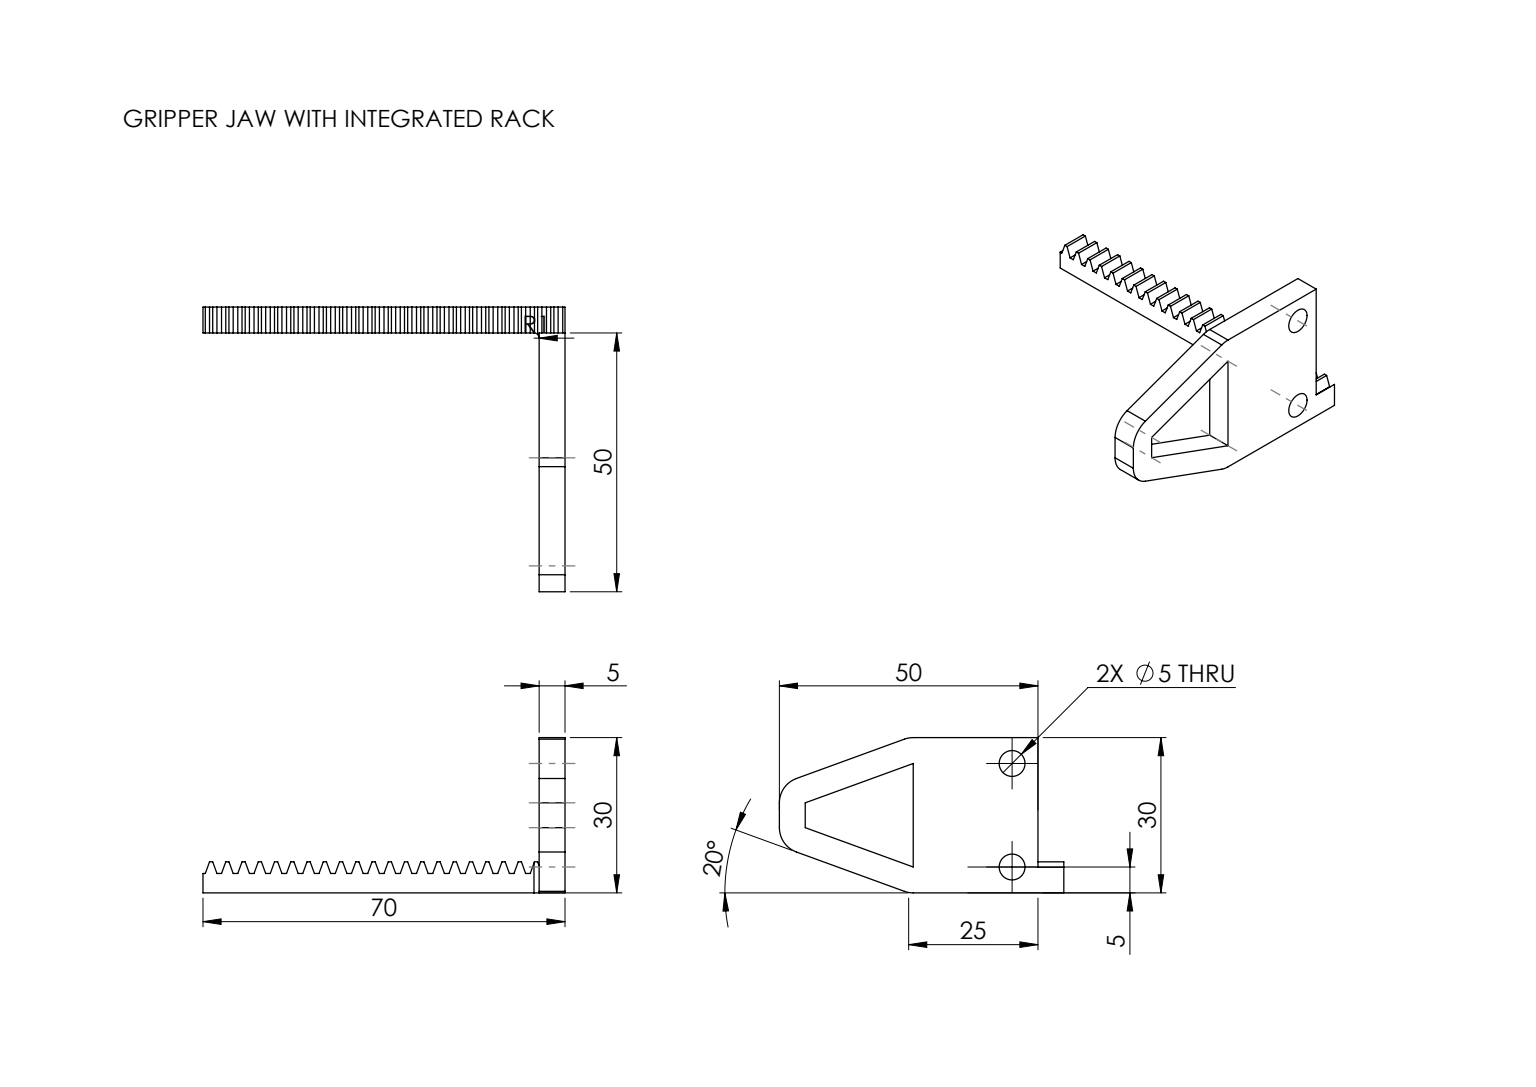
ISO-10303-21;
HEADER;
FILE_DESCRIPTION (('STEP AP214'),
    '1' );
FILE_NAME ('Gripper Jaw with Integrated Rack.step',
    '2026-10-08T13:46:47',
    ( '' ),
    ( '' ),
    'SwSTEP 2.0',
    'SolidWorks 2026',
    '' );
FILE_SCHEMA (( 'AUTOMOTIVE_DESIGN' ));
ENDSEC;

DATA;
#24=FACE_OUTER_BOUND ( 'NONE', #11980, .T. ) ;
#25=VERTEX_POINT ( 'NONE', #5216 ) ;
#26=VECTOR ( 'NONE', #20577, 1000.000000000000114 ) ;
#27=EDGE_CURVE ( 'NONE', #6815, #4177, #10288, .T. ) ;
#28=( GEOMETRIC_REPRESENTATION_CONTEXT ( 3 ) GLOBAL_UNCERTAINTY_ASSIGNED_CONTEXT ( ( #2821 ) ) GLOBAL_UNIT_ASSIGNED_CONTEXT ( ( #14742, #12246, #9459 ) ) REPRESENTATION_CONTEXT ( 'NONE', 'WORKASPACE' ) );
#29=ORIENTED_EDGE ( 'NONE', *, *, #20734, .T. ) ;
#45=ORIENTED_EDGE ( 'NONE', *, *, #7742, .T. ) ;
#53=CARTESIAN_POINT ( 'NONE',  ( 37.82128094071656932, -8.974600000000002353, 5.000000000000079936 ) ) ;
#56=LINE ( 'NONE', #21954, #15596 ) ;
#67=LINE ( 'NONE', #21968, #2877 ) ;
#70=CARTESIAN_POINT ( 'NONE',  ( -15.59503895323380362, -9.000000000000003553, 10.00000000000008882 ) ) ;
#72=ORIENTED_EDGE ( 'NONE', *, *, #3373, .F. ) ;
#76=ORIENTED_EDGE ( 'NONE', *, *, #9529, .F. ) ;
#77=LINE ( 'NONE', #11129, #17930 ) ;
#80=AXIS2_PLACEMENT_3D ( 'NONE', #20688, #15213, #18897 ) ;
#84=CARTESIAN_POINT ( 'NONE',  ( -16.41397198033274307, -11.25000000000000355, 5.000000000000079936 ) ) ;
#86=ORIENTED_EDGE ( 'NONE', *, *, #19557, .T. ) ;
#88=DIRECTION ( 'NONE',  ( 0.3420201433256622181, 0.9396926207859107594, -6.162975822039141593E-32 ) ) ;
#90=PLANE ( 'NONE',  #415 ) ;
#98=LINE ( 'NONE', #14992, #12792 ) ;
#101=DIRECTION ( 'NONE',  ( -0.9396926207859107594, -0.3420201433256623291, 1.540743955509804830E-32 ) ) ;
#102=LINE ( 'NONE', #22483, #7227 ) ;
#104=ORIENTED_EDGE ( 'NONE', *, *, #7323, .T. ) ;
#109=CARTESIAN_POINT ( 'NONE',  ( -1.594879469667249916, -11.25000000000000355, 5.000000000000079936 ) ) ;
#119=EDGE_CURVE ( 'NONE', #21784, #14801, #1618, .T. ) ;
#129=VERTEX_POINT ( 'NONE', #3181 ) ;
#134=DIRECTION ( 'NONE',  ( 0.3420201433256622736, -0.9396926207859106484, -1.232595164407828100E-31 ) ) ;
#138=ORIENTED_EDGE ( 'NONE', *, *, #22563, .F. ) ;
#156=PLANE ( 'NONE',  #640 ) ;
#163=EDGE_LOOP ( 'NONE', ( #11926, #9708, #6526, #4328 ) ) ;
#168=DIRECTION ( 'NONE',  ( 0.3420201433256622181, 0.9396926207859107594, -6.162975822039141593E-32 ) ) ;
#173=AXIS2_PLACEMENT_3D ( 'NONE', #18053, #16495, #3661 ) ;
#174=EDGE_CURVE ( 'NONE', #22879, #11902, #20401, .T. ) ;
#186=DIRECTION ( 'NONE',  ( 1.000000000000000000, 7.703719777548943412E-32, 0.000000000000000000 ) ) ;
#187=DIRECTION ( 'NONE',  ( 0.9396926207859107594, -0.3420201433256623291, 3.697785493223492838E-32 ) ) ;
#195=ORIENTED_EDGE ( 'NONE', *, *, #4034, .T. ) ;
#201=ORIENTED_EDGE ( 'NONE', *, *, #13509, .T. ) ;
#205=CARTESIAN_POINT ( 'NONE',  ( 33.85151041966726382, -11.25000000000000355, 5.000000000000079936 ) ) ;
#214=PRESENTATION_STYLE_ASSIGNMENT (( #11263 ) ) ;
#224=CARTESIAN_POINT ( 'NONE',  ( -19.99999999999999645, -9.000000000000003553, 5.000000000000079936 ) ) ;
#243=ORIENTED_EDGE ( 'NONE', *, *, #7766, .T. ) ;
#248=LINE ( 'NONE', #7582, #20083 ) ;
#270=EDGE_CURVE ( 'NONE', #13563, #6956, #18497, .T. ) ;
#275=ADVANCED_FACE ( 'NONE', ( #14703 ), #22200, .F. ) ;
#279=LINE ( 'NONE', #14812, #13339 ) ;
#280=LINE ( 'NONE', #14938, #18655 ) ;
#284=VECTOR ( 'NONE', #13283, 1000.000000000000000 ) ;
#287=AXIS2_PLACEMENT_3D ( 'NONE', #3170, #5332, #9063 ) ;
#290=FACE_OUTER_BOUND ( 'NONE', #18662, .T. ) ;
#297=VECTOR ( 'NONE', #11394, 1000.000000000000000 ) ;
#306=AXIS2_PLACEMENT_3D ( 'NONE', #17570, #1367, #5089 ) ;
#307=ORIENTED_EDGE ( 'NONE', *, *, #9563, .T. ) ;
#313=VERTEX_POINT ( 'NONE', #3887 ) ;
#327=CARTESIAN_POINT ( 'NONE',  ( 40.13469571966727045, -11.25000000000000355, 10.00000000000008882 ) ) ;
#338=VECTOR ( 'NONE', #6203, 1000.000000000000000 ) ;
#340=CARTESIAN_POINT ( 'NONE',  ( -19.99999999999999645, -9.000000000000003553, 5.000000000000079936 ) ) ;
#345=CARTESIAN_POINT ( 'NONE',  ( -4.471005642132689140, -3.347908285648603766, 10.00000000000008882 ) ) ;
#349=VECTOR ( 'NONE', #3642, 1000.000000000000000 ) ;
#353=PLANE ( 'NONE',  #2572 ) ;
#357=VECTOR ( 'NONE', #88, 1000.000000000000114 ) ;
#369=EDGE_LOOP ( 'NONE', ( #10172, #18701, #9343, #9622 ) ) ;
#371=ORIENTED_EDGE ( 'NONE', *, *, #16704, .T. ) ;
#375=VERTEX_POINT ( 'NONE', #16712 ) ;
#378=VECTOR ( 'NONE', #16810, 1000.000000000000114 ) ;
#379=VECTOR ( 'NONE', #18858, 1000.000000000000000 ) ;
#380=ORIENTED_EDGE ( 'NONE', *, *, #8945, .F. ) ;
#387=ADVANCED_FACE ( 'NONE', ( #290 ), #419, .F. ) ;
#390=CARTESIAN_POINT ( 'NONE',  ( 18.14354716966726144, -11.25000000000000355, 10.00000000000008882 ) ) ;
#394=CARTESIAN_POINT ( 'NONE',  ( 6.625378842019205905, 0.6908453745559488546, 10.00000000000008882 ) ) ;
#397=DIRECTION ( 'NONE',  ( -1.848892746611742040E-32, -0.3420201433256690460, 0.9396926207859083169 ) ) ;
#405=COLOUR_RGB ( '', 0.66274510, 0.83137255, 0.94901961) ;
#415=AXIS2_PLACEMENT_3D ( 'NONE', #22234, #2115, #9450 ) ;
#419=CYLINDRICAL_SURFACE ( 'NONE', #6270, 2.500000000000007550 ) ;
#424=EDGE_CURVE ( 'NONE', #2869, #9385, #10142, .T. ) ;
#432=ORIENTED_EDGE ( 'NONE', *, *, #13078, .F. ) ;
#435=DIRECTION ( 'NONE',  ( -0.9396926207859107594, -0.3420201433256623291, 1.540743955509804830E-32 ) ) ;
#437=DIRECTION ( 'NONE',  ( 1.000000000000000000, 7.703719777548943412E-32, 0.000000000000000000 ) ) ;
#441=EDGE_CURVE ( 'NONE', #4290, #23005, #13728, .T. ) ;
#449=ADVANCED_BREP_SHAPE_REPRESENTATION ( '', ( #22288, #7318 ), #28 ) ;
#452=EDGE_CURVE ( 'NONE', #2752, #12712, #14700, .T. ) ;
#458=EDGE_LOOP ( 'NONE', ( #20331, #17949, #19339, #14429 ) ) ;
#460=DIRECTION ( 'NONE',  ( -7.087422195345011518E-32, -1.000000000000000000, -0.000000000000000000 ) ) ;
#464=DIRECTION ( 'NONE',  ( 0.000000000000000000, 0.000000000000000000, 1.000000000000000000 ) ) ;
#469=ORIENTED_EDGE ( 'NONE', *, *, #19443, .T. ) ;
#470=LINE ( 'NONE', #15224, #23263 ) ;
#472=LINE ( 'NONE', #5983, #26 ) ;
#476=VERTEX_POINT ( 'NONE', #7853 ) ;
#483=CARTESIAN_POINT ( 'NONE',  ( 35.28529930323381336, -9.000000000000001776, 10.00000000000008882 ) ) ;
#487=LINE ( 'NONE', #7810, #20366 ) ;
#496=ORIENTED_EDGE ( 'NONE', *, *, #9040, .T. ) ;
#497=CARTESIAN_POINT ( 'NONE',  ( -19.99999999999999645, -9.000000000000003553, 5.000000000000079936 ) ) ;
#507=CARTESIAN_POINT ( 'NONE',  ( -19.55556463033274284, -11.25000000000000355, 5.000000000000079936 ) ) ;
#513=AXIS2_PLACEMENT_3D ( 'NONE', #21958, #21850, #9422 ) ;
#524=EDGE_CURVE ( 'NONE', #14801, #21630, #9665, .T. ) ;
#525=LINE ( 'NONE', #869, #679 ) ;
#526=PLANE ( 'NONE',  #15257 ) ;
#527=ORIENTED_EDGE ( 'NONE', *, *, #17288, .T. ) ;
#546=EDGE_CURVE ( 'NONE', #10073, #7680, #4255, .T. ) ;
#549=VERTEX_POINT ( 'NONE', #15298 ) ;
#557=ORIENTED_EDGE ( 'NONE', *, *, #22228, .T. ) ;
#561=DIRECTION ( 'NONE',  ( -1.000000000000000000, -7.703719777548943412E-32, 0.000000000000000000 ) ) ;
#563=LINE ( 'NONE', #5844, #11693 ) ;
#564=LINE ( 'NONE', #7663, #15899 ) ;
#575=AXIS2_PLACEMENT_3D ( 'NONE', #18890, #2475, #16877 ) ;
#576=DIRECTION ( 'NONE',  ( 0.3420201433256622181, 0.9396926207859107594, -6.162975822039141593E-32 ) ) ;
#585=EDGE_CURVE ( 'NONE', #18482, #8738, #4962, .T. ) ;
#586=CARTESIAN_POINT ( 'NONE',  ( 118.3095189484530181, -10.00000000000001599, 34.11836509645782201 ) ) ;
#592=VECTOR ( 'NONE', #4754, 1000.000000000000000 ) ;
#595=DIRECTION ( 'NONE',  ( 0.3420201433256622181, 0.9396926207859107594, -6.162975822039141593E-32 ) ) ;
#596=CARTESIAN_POINT ( 'NONE',  ( 32.14370665323380649, -9.000000000000003553, 5.000000000000079936 ) ) ;
#599=CARTESIAN_POINT ( 'NONE',  ( 44.71007725323381976, -9.000000000000003553, 5.000000000000079936 ) ) ;
#601=VECTOR ( 'NONE', #9815, 1000.000000000000000 ) ;
#602=ORIENTED_EDGE ( 'NONE', *, *, #19154, .T. ) ;
#604=EDGE_LOOP ( 'NONE', ( #19723, #19052, #12371, #5086 ) ) ;
#627=ORIENTED_EDGE ( 'NONE', *, *, #11500, .T. ) ;
#633=VERTEX_POINT ( 'NONE', #17729 ) ;
#639=EDGE_CURVE ( 'NONE', #6641, #11647, #14022, .T. ) ;
#640=AXIS2_PLACEMENT_3D ( 'NONE', #3989, #12773, #11329 ) ;
#654=CARTESIAN_POINT ( 'NONE',  ( 7.010965453233809264, -9.000000000000003553, 5.000000000000079936 ) ) ;
#664=CARTESIAN_POINT ( 'NONE',  ( 44.03180068014194148, -9.174246986850796759, 10.00000000000008704 ) ) ;
#672=CARTESIAN_POINT ( 'NONE',  ( 118.3095189484530181, 10.00000000000001599, 12.50000000000002309 ) ) ;
#675=PLANE ( 'NONE',  #14226 ) ;
#679=VECTOR ( 'NONE', #7844, 999.9999999999998863 ) ;
#682=DIRECTION ( 'NONE',  ( 0.3420201433256622181, -0.9396926207859107594, 0.000000000000000000 ) ) ;
#688=ORIENTED_EDGE ( 'NONE', *, *, #7365, .T. ) ;
#689=CARTESIAN_POINT ( 'NONE',  ( 118.3095189484530181, 10.00000000000001599, 34.11836509645782201 ) ) ;
#692=DIRECTION ( 'NONE',  ( 1.000000000000000000, 7.703719777548943412E-32, 0.000000000000000000 ) ) ;
#699=CARTESIAN_POINT ( 'NONE',  ( 40.95362874676621345, -9.000000000000003553, 5.000000000000079936 ) ) ;
#705=ORIENTED_EDGE ( 'NONE', *, *, #16420, .F. ) ;
#714=VECTOR ( 'NONE', #9364, 1000.000000000000000 ) ;
#734=AXIS2_PLACEMENT_3D ( 'NONE', #20200, #14854, #5488 ) ;
#739=AXIS2_PLACEMENT_3D ( 'NONE', #1765, #7059, #9105 ) ;
#746=CARTESIAN_POINT ( 'NONE',  ( -19.99999999999999645, -9.000000000000003553, 5.000000000000079936 ) ) ;
#750=VECTOR ( 'NONE', #3701, 1000.000000000000114 ) ;
#753=EDGE_CURVE ( 'NONE', #22275, #18422, #5493, .T. ) ;
#763=VECTOR ( 'NONE', #682, 1000.000000000000114 ) ;
#785=FACE_OUTER_BOUND ( 'NONE', #1269, .T. ) ;
#788=LINE ( 'NONE', #2452, #19506 ) ;
#796=DIRECTION ( 'NONE',  ( -1.000000000000000000, -7.703719777548943412E-32, 0.000000000000000000 ) ) ;
#813=PLANE ( 'NONE',  #14115 ) ;
#825=DIRECTION ( 'NONE',  ( 1.000000000000000000, 7.703719777548943412E-32, 0.000000000000000000 ) ) ;
#828=LINE ( 'NONE', #8044, #7240 ) ;
#833=ORIENTED_EDGE ( 'NONE', *, *, #15388, .F. ) ;
#842=EDGE_LOOP ( 'NONE', ( #23082, #13876, #7891, #7319, #20724, #21264 ) ) ;
#847=EDGE_LOOP ( 'NONE', ( #5138, #11066, #23192, #10862, #4554, #15889, #19500, #15432, #12929, #23131 ) ) ;
#868=DIRECTION ( 'NONE',  ( 1.000000000000000000, 7.703719777548943412E-32, 0.000000000000000000 ) ) ;
#869=CARTESIAN_POINT ( 'NONE',  ( 50.00000000000000000, -14.69846310392956745, 35.82846581308617573 ) ) ;
#874=ORIENTED_EDGE ( 'NONE', *, *, #14061, .F. ) ;
#877=EDGE_CURVE ( 'NONE', #11647, #2759, #4374, .T. ) ;
#879=ADVANCED_FACE ( 'NONE', ( #785 ), #15426, .F. ) ;
#890=DIRECTION ( 'NONE',  ( 0.000000000000000000, 0.000000000000000000, 1.000000000000000000 ) ) ;
#894=( NAMED_UNIT ( * ) PLANE_ANGLE_UNIT ( ) SI_UNIT ( $, .RADIAN. ) );
#896=ORIENTED_EDGE ( 'NONE', *, *, #11284, .F. ) ;
#902=CARTESIAN_POINT ( 'NONE',  ( 118.3095189484530181, -10.00000000000001954, 12.50000000000002132 ) ) ;
#903=EDGE_CURVE ( 'NONE', #10781, #17912, #2563, .T. ) ;
#915=CARTESIAN_POINT ( 'NONE',  ( 16.42649855928345204, -8.974600000000002353, 5.000000000000079936 ) ) ;
#918=CARTESIAN_POINT ( 'NONE',  ( 50.00000000000000000, 15.00000000000003375, 34.11836509645780069 ) ) ;
#920=EDGE_LOOP ( 'NONE', ( #13456, #4533, #13927, #1880 ) ) ;
#925=CARTESIAN_POINT ( 'NONE',  ( 21.28513981966725765, -11.25000000000000355, 5.000000000000079936 ) ) ;
#926=ORIENTED_EDGE ( 'NONE', *, *, #3827, .F. ) ;
#931=AXIS2_PLACEMENT_3D ( 'NONE', #13447, #6358, #11652 ) ;
#934=CARTESIAN_POINT ( 'NONE',  ( 19.57733605323380743, -9.000000000000001776, 10.00000000000008882 ) ) ;
#938=CARTESIAN_POINT ( 'NONE',  ( -19.55556463033274284, -11.25000000000000355, 10.00000000000008882 ) ) ;
#943=EDGE_CURVE ( 'NONE', #15944, #21012, #11831, .T. ) ;
#944=VECTOR ( 'NONE', #20944, 1000.000000000000114 ) ;
#951=CARTESIAN_POINT ( 'NONE',  ( -19.99999999999999645, -9.000000000000003553, 10.00000000000008882 ) ) ;
#958=EDGE_LOOP ( 'NONE', ( #20659, #18197, #9065, #7020 ) ) ;
#963=VECTOR ( 'NONE', #16673, 1000.000000000000114 ) ;
#964=DIRECTION ( 'NONE',  ( 0.3420201433256622181, 0.9396926207859107594, -6.162975822039141593E-32 ) ) ;
#965=VECTOR ( 'NONE', #15334, 1000.000000000000000 ) ;
#966=LINE ( 'NONE', #19402, #21718 ) ;
#968=CARTESIAN_POINT ( 'NONE',  ( 45.00000000000000000, -10.00000000000001954, 15.00000000000002842 ) ) ;
#974=EDGE_CURVE ( 'NONE', #20062, #17653, #8116, .T. ) ;
#983=VECTOR ( 'NONE', #15941, 1000.000000000000000 ) ;
#1001=EDGE_CURVE ( 'NONE', #4177, #4376, #17325, .T. ) ;
#1014=LINE ( 'NONE', #20885, #4918 ) ;
#1016=VERTEX_POINT ( 'NONE', #2809 ) ;
#1019=LINE ( 'NONE', #13868, #23622 ) ;
#1026=EDGE_LOOP ( 'NONE', ( #16701, #10272, #6399, #3498 ) ) ;
#1035=VERTEX_POINT ( 'NONE', #21709 ) ;
#1041=AXIS2_PLACEMENT_3D ( 'NONE', #5177, #8916, #12519 ) ;
#1045=CARTESIAN_POINT ( 'NONE',  ( -6.170261003233799890, -9.000000000000005329, 10.00000000000008882 ) ) ;
#1051=VECTOR ( 'NONE', #22738, 1000.000000000000000 ) ;
#1052=PLANE ( 'NONE',  #16049 ) ;
#1068=ADVANCED_FACE ( 'NONE', ( #5321 ), #12664, .F. ) ;
#1072=ORIENTED_EDGE ( 'NONE', *, *, #8691, .F. ) ;
#1085=LINE ( 'NONE', #4580, #2998 ) ;
#1106=ORIENTED_EDGE ( 'NONE', *, *, #11011, .F. ) ;
#1110=PLANE ( 'NONE',  #11015 ) ;
#1111=DIRECTION ( 'NONE',  ( -0.9396926207859107594, -0.3420201433256623291, 1.540743955509804830E-32 ) ) ;
#1118=AXIS2_PLACEMENT_3D ( 'NONE', #1736, #20046, #10528 ) ;
#1122=DIRECTION ( 'NONE',  ( 1.000000000000000000, 7.703719777548943412E-32, 0.000000000000000000 ) ) ;
#1124=ORIENTED_EDGE ( 'NONE', *, *, #15503, .T. ) ;
#1126=VERTEX_POINT ( 'NONE', #6891 ) ;
#1129=( GEOMETRIC_REPRESENTATION_CONTEXT ( 3 ) GLOBAL_UNCERTAINTY_ASSIGNED_CONTEXT ( ( #15787 ) ) GLOBAL_UNIT_ASSIGNED_CONTEXT ( ( #16369, #16257, #18157 ) ) REPRESENTATION_CONTEXT ( 'NONE', 'WORKASPACE' ) );
#1131=ORIENTED_EDGE ( 'NONE', *, *, #17544, .F. ) ;
#1134=DIRECTION ( 'NONE',  ( 0.000000000000000000, 0.000000000000000000, 1.000000000000000000 ) ) ;
#1142=VECTOR ( 'NONE', #15800, 1000.000000000000000 ) ;
#1151=CARTESIAN_POINT ( 'NONE',  ( 45.00000000000000000, 10.00000000000001599, 34.11836509645781490 ) ) ;
#1155=DIRECTION ( 'NONE',  ( 0.3420201433256622736, 0.9396926207859106484, 0.000000000000000000 ) ) ;
#1161=MECHANICAL_DESIGN_GEOMETRIC_PRESENTATION_REPRESENTATION('',(#6537),#4181);
#1162=EDGE_CURVE ( 'NONE', #12772, #14872, #1238, .T. ) ;
#1175=VECTOR ( 'NONE', #13412, 1000.000000000000114 ) ;
#1183=PLANE ( 'NONE',  #8483 ) ;
#1186=LINE ( 'NONE', #11771, #12491 ) ;
#1187=DIRECTION ( 'NONE',  ( 0.000000000000000000, 0.000000000000000000, 1.000000000000000000 ) ) ;
#1193=EDGE_LOOP ( 'NONE', ( #2380, #12041, #6105, #18841 ) ) ;
#1194=DIRECTION ( 'NONE',  ( 0.000000000000000000, 0.000000000000000000, -1.000000000000000000 ) ) ;
#1195=ORIENTED_EDGE ( 'NONE', *, *, #7139, .T. ) ;
#1202=EDGE_CURVE ( 'NONE', #10547, #13807, #23402, .T. ) ;
#1204=DIRECTION ( 'NONE',  ( -2.465190328815656418E-32, -0.3420201433256691015, 0.9396926207859083169 ) ) ;
#1211=ORIENTED_EDGE ( 'NONE', *, *, #17544, .T. ) ;
#1216=CARTESIAN_POINT ( 'NONE',  ( 27.56832511966726784, -11.25000000000000355, 5.000000000000079936 ) ) ;
#1218=DIRECTION ( 'NONE',  ( -1.000000000000000000, -7.703719777548943412E-32, 0.000000000000000000 ) ) ;
#1220=AXIS2_PLACEMENT_3D ( 'NONE', #17110, #4292, #7783 ) ;
#1225=LINE ( 'NONE', #8456, #17873 ) ;
#1238=LINE ( 'NONE', #1710, #19369 ) ;
#1240=EDGE_LOOP ( 'NONE', ( #9762, #18516, #602, #12286 ) ) ;
#1249=DIRECTION ( 'NONE',  ( 0.3420201433256622181, 0.9396926207859107594, -6.162975822039141593E-32 ) ) ;
#1251=DIRECTION ( 'NONE',  ( -0.9396926207859107594, -0.3420201433256623291, 1.540743955509804830E-32 ) ) ;
#1254=VECTOR ( 'NONE', #21465, 1000.000000000000000 ) ;
#1269=EDGE_LOOP ( 'NONE', ( #13649, #20440, #1072, #14194, #11128, #20415 ) ) ;
#1290=EDGE_CURVE ( 'NONE', #129, #633, #2063, .T. ) ;
#1298=CARTESIAN_POINT ( 'NONE',  ( -18.73663160323380339, -9.000000000000003553, 5.000000000000079936 ) ) ;
#1300=AXIS2_PLACEMENT_3D ( 'NONE', #4873, #10299, #6568 ) ;
#1302=ADVANCED_FACE ( 'NONE', ( #23641 ), #156, .F. ) ;
#1307=DIRECTION ( 'NONE',  ( -0.3420201433256622181, 0.9396926207859106484, 1.232595164407828100E-31 ) ) ;
#1324=CARTESIAN_POINT ( 'NONE',  ( -10.13078668033273999, -11.25000000000000355, 5.000000000000079936 ) ) ;
#1327=ORIENTED_EDGE ( 'NONE', *, *, #6855, .T. ) ;
#1352=VECTOR ( 'NONE', #12908, 1000.000000000000000 ) ;
#1364=ORIENTED_EDGE ( 'NONE', *, *, #4274, .T. ) ;
#1367=DIRECTION ( 'NONE',  ( -1.000000000000000000, -7.703719777548943412E-32, 0.000000000000000000 ) ) ;
#1370=DIRECTION ( 'NONE',  ( 0.000000000000000000, 0.000000000000000000, -1.000000000000000000 ) ) ;
#1378=LINE ( 'NONE', #19478, #2861 ) ;
#1380=EDGE_LOOP ( 'NONE', ( #22643, #4683, #7458, #15884 ) ) ;
#1383=FACE_OUTER_BOUND ( 'NONE', #10306, .T. ) ;
#1386=CARTESIAN_POINT ( 'NONE',  ( 3.263761790716562139, -8.974600000000002353, 5.000000000000079936 ) ) ;
#1389=DIRECTION ( 'NONE',  ( 1.000000000000000000, 7.703719777548943412E-32, 0.000000000000000000 ) ) ;
#1394=CARTESIAN_POINT ( 'NONE',  ( 28.39650299071657003, -8.974600000000002353, 5.000000000000079936 ) ) ;
#1400=PLANE ( 'NONE',  #4170 ) ;
#1421=ORIENTED_EDGE ( 'NONE', *, *, #7801, .T. ) ;
#1427=EDGE_CURVE ( 'NONE', #12772, #21867, #14168, .T. ) ;
#1433=LINE ( 'NONE', #8656, #7623 ) ;
#1441=FACE_OUTER_BOUND ( 'NONE', #20684, .T. ) ;
#1463=DIRECTION ( 'NONE',  ( -0.3420201433256622181, 0.9396926207859106484, 1.232595164407828100E-31 ) ) ;
#1477=VECTOR ( 'NONE', #3706, 1000.000000000000000 ) ;
#1481=ORIENTED_EDGE ( 'NONE', *, *, #22334, .F. ) ;
#1484=DIRECTION ( 'NONE',  ( 0.3420201433256622736, -0.9396926207859106484, -1.232595164407828100E-31 ) ) ;
#1485=ORIENTED_EDGE ( 'NONE', *, *, #10165, .T. ) ;
#1497=ORIENTED_EDGE ( 'NONE', *, *, #22701, .T. ) ;
#1502=EDGE_CURVE ( 'NONE', #11449, #21785, #7339, .T. ) ;
#1522=ORIENTED_EDGE ( 'NONE', *, *, #14669, .T. ) ;
#1532=CARTESIAN_POINT ( 'NONE',  ( 22.70968385928345157, -8.974600000000002353, 5.000000000000079936 ) ) ;
#1544=EDGE_CURVE ( 'NONE', #8315, #18533, #3361, .T. ) ;
#1547=CARTESIAN_POINT ( 'NONE',  ( 31.53809564071656624, -8.974600000000002353, 10.00000000000008882 ) ) ;
#1550=VERTEX_POINT ( 'NONE', #8895 ) ;
#1558=DIRECTION ( 'NONE',  ( 0.000000000000000000, 0.000000000000000000, 1.000000000000000000 ) ) ;
#1560=LINE ( 'NONE', #9021, #16034 ) ;
#1564=DIRECTION ( 'NONE',  ( 0.3420201433256622181, -0.9396926207859107594, 0.000000000000000000 ) ) ;
#1571=ORIENTED_EDGE ( 'NONE', *, *, #13112, .T. ) ;
#1575=ADVANCED_FACE ( 'NONE', ( #3592 ), #21669, .T. ) ;
#1577=ORIENTED_EDGE ( 'NONE', *, *, #12655, .F. ) ;
#1578=CARTESIAN_POINT ( 'NONE',  ( -18.34148624732256394, -8.396350360904289545, 10.00000000000008882 ) ) ;
#1579=ORIENTED_EDGE ( 'NONE', *, *, #22022, .F. ) ;
#1581=EDGE_LOOP ( 'NONE', ( #527, #11428, #15379, #1485 ) ) ;
#1605=ORIENTED_EDGE ( 'NONE', *, *, #16420, .T. ) ;
#1618=LINE ( 'NONE', #7150, #16240 ) ;
#1629=LINE ( 'NONE', #8603, #18204 ) ;
#1646=FACE_OUTER_BOUND ( 'NONE', #13158, .T. ) ;
#1647=ORIENTED_EDGE ( 'NONE', *, *, #13509, .F. ) ;
#1649=CARTESIAN_POINT ( 'NONE',  ( -19.99999999999999645, -9.000000000000003553, 10.00000000000008882 ) ) ;
#1657=VECTOR ( 'NONE', #15828, 1000.000000000000114 ) ;
#1660=DIRECTION ( 'NONE',  ( 0.000000000000000000, 0.000000000000000000, -1.000000000000000000 ) ) ;
#1667=CARTESIAN_POINT ( 'NONE',  ( 6.396109596766199168, -9.000000000000005329, 10.00000000000008882 ) ) ;
#1669=LINE ( 'NONE', #17740, #23238 ) ;
#1673=LINE ( 'NONE', #21900, #11101 ) ;
#1674=DIRECTION ( 'NONE',  ( 1.000000000000000000, 7.703719777548943412E-32, 0.000000000000000000 ) ) ;
#1679=FACE_OUTER_BOUND ( 'NONE', #7171, .T. ) ;
#1685=ORIENTED_EDGE ( 'NONE', *, *, #1427, .T. ) ;
#1687=EDGE_LOOP ( 'NONE', ( #9119, #10883, #469, #20663 ) ) ;
#1692=EDGE_LOOP ( 'NONE', ( #12643, #19226, #4435, #11190 ) ) ;
#1707=ADVANCED_FACE ( 'NONE', ( #23509 ), #21828, .F. ) ;
#1710=CARTESIAN_POINT ( 'NONE',  ( 43.27628836966725601, -11.25000000000000355, 5.000000000000079936 ) ) ;
#1718=LINE ( 'NONE', #14330, #19683 ) ;
#1721=ORIENTED_EDGE ( 'NONE', *, *, #639, .F. ) ;
#1736=CARTESIAN_POINT ( 'NONE',  ( 46.41788101966725577, -11.25000000000000355, 5.000000000000079936 ) ) ;
#1745=DIRECTION ( 'NONE',  ( -0.9396926207859107594, -0.3420201433256623291, 1.540743955509804830E-32 ) ) ;
#1754=ORIENTED_EDGE ( 'NONE', *, *, #4128, .F. ) ;
#1759=LINE ( 'NONE', #21873, #20990 ) ;
#1763=EDGE_LOOP ( 'NONE', ( #23490, #23359, #7432, #18985 ) ) ;
#1765=CARTESIAN_POINT ( 'NONE',  ( -19.99999999999999645, -9.000000000000003553, 5.000000000000079936 ) ) ;
#1768=DIRECTION ( 'NONE',  ( 7.200064461366508930E-32, 1.000000000000000000, 5.754033390038004481E-16 ) ) ;
#1777=CARTESIAN_POINT ( 'NONE',  ( -19.99999999999999645, -9.000000000000003553, 5.000000000000079936 ) ) ;
#1783=ORIENTED_EDGE ( 'NONE', *, *, #5073, .T. ) ;
#1786=CARTESIAN_POINT ( 'NONE',  ( 45.00000000000000000, -7.098169556225942145, 56.71010071662853136 ) ) ;
#1811=VECTOR ( 'NONE', #23079, 1000.000000000000000 ) ;
#1823=VECTOR ( 'NONE', #6635, 1000.000000000000114 ) ;
#1827=ORIENTED_EDGE ( 'NONE', *, *, #23114, .T. ) ;
#1835=VERTEX_POINT ( 'NONE', #7480 ) ;
#1839=CARTESIAN_POINT ( 'NONE',  ( 27.56832511966726784, -11.25000000000000355, 5.000000000000079936 ) ) ;
#1843=CARTESIAN_POINT ( 'NONE',  ( 45.00000000000000000, -14.69846310392956745, 35.82846581308617573 ) ) ;
#1853=FACE_OUTER_BOUND ( 'NONE', #22121, .T. ) ;
#1856=VERTEX_POINT ( 'NONE', #16932 ) ;
#1859=PLANE ( 'NONE',  #18241 ) ;
#1871=VECTOR ( 'NONE', #9335, 1000.000000000000000 ) ;
#1878=CARTESIAN_POINT ( 'NONE',  ( 118.3095189484530181, 7.098169556225943033, 56.71010071662853136 ) ) ;
#1880=ORIENTED_EDGE ( 'NONE', *, *, #23008, .T. ) ;
#1887=CARTESIAN_POINT ( 'NONE',  ( 32.13446180928345086, -8.974600000000002353, 5.000000000000079936 ) ) ;
#1909=CIRCLE ( 'NONE', #4587, 2.500000000000007550 ) ;
#1935=ADVANCED_FACE ( 'NONE', ( #15270 ), #2532, .F. ) ;
#1942=CARTESIAN_POINT ( 'NONE',  ( 13.29415075323381323, -9.000000000000001776, 5.000000000000079936 ) ) ;
#1948=CARTESIAN_POINT ( 'NONE',  ( 50.00000000000000000, -2.399706452296352932, 60.00000000000021316 ) ) ;
#1956=ORIENTED_EDGE ( 'NONE', *, *, #18593, .T. ) ;
#1959=LINE ( 'NONE', #5447, #11042 ) ;
#1977=LINE ( 'NONE', #5353, #6317 ) ;
#1980=DIRECTION ( 'NONE',  ( 0.000000000000000000, 0.000000000000000000, 1.000000000000000000 ) ) ;
#1981=VERTEX_POINT ( 'NONE', #13582 ) ;
#1989=LINE ( 'NONE', #20550, #20553 ) ;
#1990=EDGE_LOOP ( 'NONE', ( #6524, #5819, #17095, #15250 ) ) ;
#1993=CARTESIAN_POINT ( 'NONE',  ( -3.028668353233801458, -9.000000000000005329, 5.000000000000079936 ) ) ;
#1996=DIRECTION ( 'NONE',  ( 0.000000000000000000, 0.000000000000000000, -1.000000000000000000 ) ) ;
#2004=SURFACE_STYLE_FILL_AREA ( #5852 ) ;
#2021=VECTOR ( 'NONE', #22689, 1000.000000000000000 ) ;
#2037=ADVANCED_FACE ( 'NONE', ( #13351 ), #19066, .T. ) ;
#2040=ORIENTED_EDGE ( 'NONE', *, *, #16782, .T. ) ;
#2043=DIRECTION ( 'NONE',  ( 0.000000000000000000, 0.000000000000000000, 1.000000000000000000 ) ) ;
#2044=VERTEX_POINT ( 'NONE', #6262 ) ;
#2046=CARTESIAN_POINT ( 'NONE',  ( 24.42673246966726452, -11.25000000000000355, 5.000000000000079936 ) ) ;
#2052=PLANE ( 'NONE',  #11510 ) ;
#2060=DIRECTION ( 'NONE',  ( 0.000000000000000000, 0.000000000000000000, 1.000000000000000000 ) ) ;
#2063=LINE ( 'NONE', #14684, #18233 ) ;
#2070=ORIENTED_EDGE ( 'NONE', *, *, #7765, .F. ) ;
#2089=CARTESIAN_POINT ( 'NONE',  ( -9.311853653233802319, -9.000000000000003553, 5.000000000000079936 ) ) ;
#2092=ORIENTED_EDGE ( 'NONE', *, *, #15142, .F. ) ;
#2113=CARTESIAN_POINT ( 'NONE',  ( 0.1129242967662022479, -9.000000000000001776, 10.00000000000008882 ) ) ;
#2115=DIRECTION ( 'NONE',  ( -0.9396926207859107594, -0.3420201433256623291, 1.540743955509804830E-32 ) ) ;
#2116=DIRECTION ( 'NONE',  ( 0.3420201433256622181, -0.9396926207859107594, 0.000000000000000000 ) ) ;
#2128=FACE_OUTER_BOUND ( 'NONE', #8630, .T. ) ;
#2131=VERTEX_POINT ( 'NONE', #3129 ) ;
#2135=CARTESIAN_POINT ( 'NONE',  ( 26.67945438033275707, -11.25000000000000355, 10.00000000000008882 ) ) ;
#2139=LINE ( 'NONE', #4067, #20538 ) ;
#2160=DIRECTION ( 'NONE',  ( 0.000000000000000000, 0.000000000000000000, 1.000000000000000000 ) ) ;
#2196=CARTESIAN_POINT ( 'NONE',  ( 39.24582498033275613, -11.25000000000000355, 10.00000000000008882 ) ) ;
#2197=EDGE_CURVE ( 'NONE', #20481, #6488, #23638, .T. ) ;
#2198=DIRECTION ( 'NONE',  ( -0.3420201433256622181, 0.9396926207859106484, 1.232595164407828100E-31 ) ) ;
#2200=VECTOR ( 'NONE', #14134, 1000.000000000000000 ) ;
#2206=DIRECTION ( 'NONE',  ( 0.000000000000000000, 0.000000000000000000, 1.000000000000000000 ) ) ;
#2207=LINE ( 'NONE', #20162, #379 ) ;
#2229=EDGE_CURVE ( 'NONE', #23499, #10887, #14567, .T. ) ;
#2265=DIRECTION ( 'NONE',  ( 0.3420201433256622181, 0.9396926207859107594, -6.162975822039141593E-32 ) ) ;
#2266=DIRECTION ( 'NONE',  ( 0.3420201433256622736, 0.9396926207859106484, 0.000000000000000000 ) ) ;
#2268=AXIS2_PLACEMENT_3D ( 'NONE', #1394, #16277, #8988 ) ;
#2276=LINE ( 'NONE', #17019, #23504 ) ;
#2284=ORIENTED_EDGE ( 'NONE', *, *, #17458, .F. ) ;
#2286=EDGE_LOOP ( 'NONE', ( #2477, #16579, #11571, #7358 ) ) ;
#2292=ORIENTED_EDGE ( 'NONE', *, *, #13935, .T. ) ;
#2295=ORIENTED_EDGE ( 'NONE', *, *, #5529, .T. ) ;
#2300=VECTOR ( 'NONE', #14417, 1000.000000000000000 ) ;
#2312=DIRECTION ( 'NONE',  ( -7.087422195345011518E-32, -1.000000000000000000, 0.000000000000000000 ) ) ;
#2321=ORIENTED_EDGE ( 'NONE', *, *, #20642, .F. ) ;
#2337=DIRECTION ( 'NONE',  ( 0.000000000000000000, 0.000000000000000000, -1.000000000000000000 ) ) ;
#2345=VERTEX_POINT ( 'NONE', #17498 ) ;
#2354=DIRECTION ( 'NONE',  ( -1.000000000000000000, -7.703719777548943412E-32, 0.000000000000000000 ) ) ;
#2366=VERTEX_POINT ( 'NONE', #13451 ) ;
#2371=EDGE_CURVE ( 'NONE', #14828, #6681, #13805, .T. ) ;
#2374=DIRECTION ( 'NONE',  ( 0.000000000000000000, 0.000000000000000000, -1.000000000000000000 ) ) ;
#2375=DIRECTION ( 'NONE',  ( 1.000000000000000000, 7.703719777548943412E-32, 0.000000000000000000 ) ) ;
#2380=ORIENTED_EDGE ( 'NONE', *, *, #4128, .T. ) ;
#2385=CARTESIAN_POINT ( 'NONE',  ( 40.96287359071656908, -8.974600000000002353, 5.000000000000079936 ) ) ;
#2398=PLANE ( 'NONE',  #23329 ) ;
#2408=VERTEX_POINT ( 'NONE', #13678 ) ;
#2409=ORIENTED_EDGE ( 'NONE', *, *, #10292, .F. ) ;
#2417=DIRECTION ( 'NONE',  ( 0.000000000000000000, 0.000000000000000000, -1.000000000000000000 ) ) ;
#2433=DIRECTION ( 'NONE',  ( 7.087422195345011518E-32, 1.000000000000000000, 0.000000000000000000 ) ) ;
#2444=CARTESIAN_POINT ( 'NONE',  ( 9.537702246766199821, -9.000000000000005329, 5.000000000000079936 ) ) ;
#2448=DIRECTION ( 'NONE',  ( 0.3420201433256622181, -0.9396926207859107594, 0.000000000000000000 ) ) ;
#2452=CARTESIAN_POINT ( 'NONE',  ( 3.869372803233808611, -9.000000000000003553, 5.000000000000079936 ) ) ;
#2457=CARTESIAN_POINT ( 'NONE',  ( 15.00195451966726523, -11.25000000000000355, 5.000000000000079936 ) ) ;
#2461=EDGE_CURVE ( 'NONE', #2366, #11492, #17025, .T. ) ;
#2464=VECTOR ( 'NONE', #9085, 1000.000000000000000 ) ;
#2470=EDGE_CURVE ( 'NONE', #12570, #16559, #7071, .T. ) ;
#2475=DIRECTION ( 'NONE',  ( -0.9396926207859107594, -0.3420201433256623291, 1.540743955509804830E-32 ) ) ;
#2477=ORIENTED_EDGE ( 'NONE', *, *, #19719, .T. ) ;
#2481=DIRECTION ( 'NONE',  ( 1.000000000000000000, 7.703719777548943412E-32, 0.000000000000000000 ) ) ;
#2483=LINE ( 'NONE', #10064, #17040 ) ;
#2486=VECTOR ( 'NONE', #9908, 1000.000000000000000 ) ;
#2523=EDGE_LOOP ( 'NONE', ( #11872, #13867, #11518, #21273 ) ) ;
#2528=EDGE_CURVE ( 'NONE', #4844, #5170, #10805, .T. ) ;
#2532=PLANE ( 'NONE',  #5477 ) ;
#2546=DIRECTION ( 'NONE',  ( -1.000000000000000000, -7.703719777548943412E-32, 0.000000000000000000 ) ) ;
#2547=ORIENTED_EDGE ( 'NONE', *, *, #21664, .F. ) ;
#2556=LINE ( 'NONE', #9904, #5357 ) ;
#2563=LINE ( 'NONE', #9910, #22680 ) ;
#2566=CARTESIAN_POINT ( 'NONE',  ( 118.3095189484530181, 14.69846310392956745, 35.82846581308617573 ) ) ;
#2572=AXIS2_PLACEMENT_3D ( 'NONE', #7687, #15005, #2266 ) ;
#2578=VECTOR ( 'NONE', #1980, 1000.000000000000000 ) ;
#2590=CARTESIAN_POINT ( 'NONE',  ( 50.00000000000000000, -10.00000000000001599, 34.11836509645782201 ) ) ;
#2594=CYLINDRICAL_SURFACE ( 'NONE', #1300, 2.500000000000007550 ) ;
#2598=FACE_OUTER_BOUND ( 'NONE', #23227, .T. ) ;
#2599=LINE ( 'NONE', #19007, #14646 ) ;
#2607=DIRECTION ( 'NONE',  ( 1.000000000000000000, 7.703719777548943412E-32, 0.000000000000000000 ) ) ;
#2611=CARTESIAN_POINT ( 'NONE',  ( 35.27605445928345063, -8.974600000000002353, 5.000000000000079936 ) ) ;
#2618=ORIENTED_EDGE ( 'NONE', *, *, #7801, .F. ) ;
#2620=EDGE_CURVE ( 'NONE', #6127, #11172, #14510, .T. ) ;
#2626=VECTOR ( 'NONE', #4607, 1000.000000000000000 ) ;
#2627=LINE ( 'NONE', #596, #20681 ) ;
#2639=VECTOR ( 'NONE', #1564, 1000.000000000000114 ) ;
#2644=EDGE_CURVE ( 'NONE', #21534, #19492, #98, .T. ) ;
#2658=DIRECTION ( 'NONE',  ( 0.000000000000000000, 0.000000000000000000, 1.000000000000000000 ) ) ;
#2662=VECTOR ( 'NONE', #10669, 1000.000000000000114 ) ;
#2674=VECTOR ( 'NONE', #18506, 1000.000000000000000 ) ;
#2690=VECTOR ( 'NONE', #8286, 1000.000000000000000 ) ;
#2702=VERTEX_POINT ( 'NONE', #12723 ) ;
#2703=DIRECTION ( 'NONE',  ( 0.000000000000000000, 0.000000000000000000, 1.000000000000000000 ) ) ;
#2711=EDGE_LOOP ( 'NONE', ( #2739, #10483, #7158, #19964 ) ) ;
#2714=DIRECTION ( 'NONE',  ( 0.3420201433256622736, -0.9396926207859106484, -1.232595164407828100E-31 ) ) ;
#2724=EDGE_LOOP ( 'NONE', ( #4740, #22610, #2547, #23003 ) ) ;
#2729=VERTEX_POINT ( 'NONE', #5614 ) ;
#2735=DIRECTION ( 'NONE',  ( 7.087422195345011518E-32, 1.000000000000000000, -0.000000000000000000 ) ) ;
#2739=ORIENTED_EDGE ( 'NONE', *, *, #16134, .T. ) ;
#2745=DIRECTION ( 'NONE',  ( 0.000000000000000000, 0.000000000000000000, 1.000000000000000000 ) ) ;
#2752=VERTEX_POINT ( 'NONE', #22117 ) ;
#2756=ORIENTED_EDGE ( 'NONE', *, *, #12561, .F. ) ;
#2759=VERTEX_POINT ( 'NONE', #16522 ) ;
#2763=LINE ( 'NONE', #19179, #20522 ) ;
#2784=VERTEX_POINT ( 'NONE', #9701 ) ;
#2789=DIRECTION ( 'NONE',  ( 0.3420201433256622736, 0.9396926207859106484, 0.000000000000000000 ) ) ;
#2793=ADVANCED_FACE ( 'NONE', ( #13422 ), #15339, .T. ) ;
#2796=EDGE_CURVE ( 'NONE', #10456, #15720, #20343, .T. ) ;
#2809=CARTESIAN_POINT ( 'NONE',  ( 32.96263968033274949, -11.25000000000000355, 5.000000000000079936 ) ) ;
#2814=ORIENTED_EDGE ( 'NONE', *, *, #424, .T. ) ;
#2821=UNCERTAINTY_MEASURE_WITH_UNIT (LENGTH_MEASURE( 1.000000000000000082E-05 ), #14742, 'distance_accuracy_value', 'NONE');
#2824=EDGE_CURVE ( 'NONE', #7050, #8315, #2599, .T. ) ;
#2826=FACE_OUTER_BOUND ( 'NONE', #1763, .T. ) ;
#2834=CARTESIAN_POINT ( 'NONE',  ( -13.27237933033274153, -11.25000000000000355, 5.000000000000079936 ) ) ;
#2837=LINE ( 'NONE', #6576, #23549 ) ;
#2839=DIRECTION ( 'NONE',  ( -0.9396926207859107594, -0.3420201433256623291, 1.540743955509804830E-32 ) ) ;
#2840=ORIENTED_EDGE ( 'NONE', *, *, #174, .T. ) ;
#2856=VECTOR ( 'NONE', #23217, 1000.000000000000000 ) ;
#2857=DIRECTION ( 'NONE',  ( 0.000000000000000000, 0.000000000000000000, 1.000000000000000000 ) ) ;
#2858=ORIENTED_EDGE ( 'NONE', *, *, #16088, .F. ) ;
#2861=VECTOR ( 'NONE', #10419, 1000.000000000000114 ) ;
#2866=DIRECTION ( 'NONE',  ( 0.3420201433256622736, 0.9396926207859106484, 0.000000000000000000 ) ) ;
#2869=VERTEX_POINT ( 'NONE', #16997 ) ;
#2870=LINE ( 'NONE', #20948, #21606 ) ;
#2877=VECTOR ( 'NONE', #4018, 1000.000000000000000 ) ;
#2900=ORIENTED_EDGE ( 'NONE', *, *, #5899, .T. ) ;
#2907=FACE_OUTER_BOUND ( 'NONE', #13297, .T. ) ;
#2914=EDGE_CURVE ( 'NONE', #6569, #13807, #4525, .T. ) ;
#2919=VERTEX_POINT ( 'NONE', #6088 ) ;
#2922=ORIENTED_EDGE ( 'NONE', *, *, #11454, .F. ) ;
#2927=EDGE_LOOP ( 'NONE', ( #23459, #5244, #12916, #5062 ) ) ;
#2933=CARTESIAN_POINT ( 'NONE',  ( -16.41397198033274307, -11.25000000000000355, 5.000000000000079936 ) ) ;
#2934=EDGE_CURVE ( 'NONE', #10781, #21477, #15575, .T. ) ;
#2936=VECTOR ( 'NONE', #23113, 1000.000000000000000 ) ;
#2947=CARTESIAN_POINT ( 'NONE',  ( -8.696997796766190447, -9.000000000000005329, 10.00000000000008882 ) ) ;
#2955=ADVANCED_FACE ( 'NONE', ( #21031 ), #19245, .F. ) ;
#2959=EDGE_LOOP ( 'NONE', ( #76, #17152, #20067, #4280 ) ) ;
#2963=VECTOR ( 'NONE', #21400, 1000.000000000000000 ) ;
#2964=CARTESIAN_POINT ( 'NONE',  ( 50.00000000000000000, 10.00000000000001599, 34.11836509645782201 ) ) ;
#2996=PRODUCT_DEFINITION ( 'UNKNOWN', '', #17578, #4530 ) ;
#2998=VECTOR ( 'NONE', #12138, 1000.000000000000000 ) ;
#3018=ORIENTED_EDGE ( 'NONE', *, *, #14669, .F. ) ;
#3047=CARTESIAN_POINT ( 'NONE',  ( 0.1221691407165617638, -8.974600000000002353, 5.000000000000079936 ) ) ;
#3051=( NAMED_UNIT ( * ) SI_UNIT ( $, .STERADIAN. ) SOLID_ANGLE_UNIT ( ) );
#3052=VECTOR ( 'NONE', #20998, 1000.000000000000000 ) ;
#3054=ORIENTED_EDGE ( 'NONE', *, *, #6171, .F. ) ;
#3067=VECTOR ( 'NONE', #19537, 1000.000000000000000 ) ;
#3081=CARTESIAN_POINT ( 'NONE',  ( 40.13469571966727045, -11.25000000000000355, 5.000000000000079936 ) ) ;
#3083=VECTOR ( 'NONE', #13544, 1000.000000000000000 ) ;
#3090=ORIENTED_EDGE ( 'NONE', *, *, #3478, .T. ) ;
#3111=CARTESIAN_POINT ( 'NONE',  ( 0.000000000000000000, 0.000000000000000000, 0.000000000000000000 ) ) ;
#3118=ORIENTED_EDGE ( 'NONE', *, *, #10409, .F. ) ;
#3120=EDGE_LOOP ( 'NONE', ( #8165, #22127, #18181, #17207 ) ) ;
#3122=CARTESIAN_POINT ( 'NONE',  ( 0.1221691407165617638, -8.974600000000002353, 10.00000000000008882 ) ) ;
#3128=ADVANCED_FACE ( 'NONE', ( #1383 ), #16030, .F. ) ;
#3129=CARTESIAN_POINT ( 'NONE',  ( 28.38725814676620018, -9.000000000000007105, 10.00000000000008882 ) ) ;
#3132=CARTESIAN_POINT ( 'NONE',  ( 45.00000000000000000, -9.796556200126357083, 11.00000000000008882 ) ) ;
#3134=ORIENTED_EDGE ( 'NONE', *, *, #1290, .T. ) ;
#3142=ORIENTED_EDGE ( 'NONE', *, *, #12124, .F. ) ;
#3149=CARTESIAN_POINT ( 'NONE',  ( 45.00000000000000000, -10.00000000000001954, 15.00000000000002842 ) ) ;
#3158=ORIENTED_EDGE ( 'NONE', *, *, #11859, .T. ) ;
#3159=CARTESIAN_POINT ( 'NONE',  ( 3.263761790716562139, -8.974600000000002353, 10.00000000000008882 ) ) ;
#3166=EDGE_LOOP ( 'NONE', ( #1522, #12488, #16609, #3193 ) ) ;
#3167=EDGE_LOOP ( 'NONE', ( #14963, #4236, #3384, #15830 ) ) ;
#3169=EDGE_CURVE ( 'NONE', #3905, #11172, #20295, .T. ) ;
#3170=CARTESIAN_POINT ( 'NONE',  ( -6.989194030332740226, -11.25000000000000355, 5.000000000000079936 ) ) ;
#3171=LINE ( 'NONE', #12076, #22088 ) ;
#3172=VERTEX_POINT ( 'NONE', #14715 ) ;
#3174=LINE ( 'NONE', #19020, #6016 ) ;
#3181=CARTESIAN_POINT ( 'NONE',  ( 44.09522139676619901, -9.000000000000003553, 10.00454388062671640 ) ) ;
#3186=CARTESIAN_POINT ( 'NONE',  ( 27.56832511966726784, -11.25000000000000355, 10.00000000000008882 ) ) ;
#3187=VECTOR ( 'NONE', #12322, 1000.000000000000114 ) ;
#3193=ORIENTED_EDGE ( 'NONE', *, *, #20000, .T. ) ;
#3197=ADVANCED_FACE ( 'NONE', ( #14600 ), #5467, .T. ) ;
#3207=FACE_OUTER_BOUND ( 'NONE', #3469, .T. ) ;
#3220=EDGE_CURVE ( 'NONE', #3825, #18250, #1977, .T. ) ;
#3221=CARTESIAN_POINT ( 'NONE',  ( -15.58579410928343911, -8.974600000000002353, 5.000000000000079936 ) ) ;
#3229=ORIENTED_EDGE ( 'NONE', *, *, #13078, .T. ) ;
#3248=CARTESIAN_POINT ( 'NONE',  ( -17.30284271966725029, -11.25000000000000355, 5.000000000000079936 ) ) ;
#3266=ADVANCED_FACE ( 'NONE', ( #3900 ), #18164, .T. ) ;
#3268=ADVANCED_FACE ( 'NONE', ( #18398 ), #13037, .F. ) ;
#3270=CARTESIAN_POINT ( 'NONE',  ( 36.99310306966726358, -11.25000000000000355, 5.000000000000079936 ) ) ;
#3279=VECTOR ( 'NONE', #16962, 1000.000000000000114 ) ;
#3290=FACE_OUTER_BOUND ( 'NONE', #8292, .T. ) ;
#3306=SURFACE_STYLE_FILL_AREA ( #19702 ) ;
#3308=CARTESIAN_POINT ( 'NONE',  ( -18.73663160323380339, -9.000000000000003553, 10.00000000000008882 ) ) ;
#3335=VECTOR ( 'NONE', #2703, 1000.000000000000000 ) ;
#3337=LINE ( 'NONE', #5025, #5924 ) ;
#3339=LINE ( 'NONE', #21528, #20284 ) ;
#3340=EDGE_LOOP ( 'NONE', ( #4442, #9333, #23525, #23681 ) ) ;
#3347=PLANE ( 'NONE',  #14370 ) ;
#3349=DIRECTION ( 'NONE',  ( 0.3420201433256622181, 0.9396926207859107594, -6.162975822039141593E-32 ) ) ;
#3354=ORIENTED_EDGE ( 'NONE', *, *, #3511, .T. ) ;
#3361=LINE ( 'NONE', #8653, #12140 ) ;
#3368=FACE_OUTER_BOUND ( 'NONE', #10344, .T. ) ;
#3373=EDGE_CURVE ( 'NONE', #13272, #19009, #23353, .T. ) ;
#3374=ORIENTED_EDGE ( 'NONE', *, *, #15548, .T. ) ;
#3384=ORIENTED_EDGE ( 'NONE', *, *, #20801, .F. ) ;
#3389=CARTESIAN_POINT ( 'NONE',  ( -11.01965741966725076, -11.25000000000000355, 10.00000000000008882 ) ) ;
#3390=LINE ( 'NONE', #21457, #12606 ) ;
#3401=EDGE_CURVE ( 'NONE', #10887, #19450, #14393, .T. ) ;
#3410=EDGE_LOOP ( 'NONE', ( #6581, #15026, #15750, #833, #17567, #4157, #18580, #9790, #6032, #3054, #8869, #4896 ) ) ;
#3415=VECTOR ( 'NONE', #12382, 1000.000000000000000 ) ;
#3428=VECTOR ( 'NONE', #2448, 1000.000000000000114 ) ;
#3431=PLANE ( 'NONE',  #7637 ) ;
#3439=ORIENTED_EDGE ( 'NONE', *, *, #11322, .T. ) ;
#3444=EDGE_LOOP ( 'NONE', ( #13156, #7205, #11208, #12331 ) ) ;
#3446=EDGE_LOOP ( 'NONE', ( #18459, #7578, #16120, #14007 ) ) ;
#3469=EDGE_LOOP ( 'NONE', ( #138, #11067, #4937, #19301 ) ) ;
#3478=EDGE_CURVE ( 'NONE', #22731, #313, #10811, .T. ) ;
#3487=CARTESIAN_POINT ( 'NONE',  ( -19.99999999999999645, -9.000000000000003553, 5.000000000000079936 ) ) ;
#3498=ORIENTED_EDGE ( 'NONE', *, *, #21456, .T. ) ;
#3511=EDGE_CURVE ( 'NONE', #15223, #25, #12728, .T. ) ;
#3520=CARTESIAN_POINT ( 'NONE',  ( 25.24566549676620397, -9.000000000000003553, 5.000000000000079936 ) ) ;
#3523=CARTESIAN_POINT ( 'NONE',  ( -19.99999999999999645, -9.000000000000003553, 5.000000000000079936 ) ) ;
#3564=LINE ( 'NONE', #5481, #6043 ) ;
#3565=CARTESIAN_POINT ( 'NONE',  ( -13.27237933033274153, -11.25000000000000355, 5.000000000000079936 ) ) ;
#3581=FACE_OUTER_BOUND ( 'NONE', #6661, .T. ) ;
#3583=CARTESIAN_POINT ( 'NONE',  ( -19.55556463033274284, -11.25000000000000355, 5.000000000000079936 ) ) ;
#3591=CARTESIAN_POINT ( 'NONE',  ( -19.99999999999999645, -9.000000000000003553, 10.00000000000008882 ) ) ;
#3592=FACE_OUTER_BOUND ( 'NONE', #6776, .T. ) ;
#3602=ORIENTED_EDGE ( 'NONE', *, *, #11998, .F. ) ;
#3604=EDGE_LOOP ( 'NONE', ( #1577, #4463, #18161, #11524 ) ) ;
#3632=AXIS2_PLACEMENT_3D ( 'NONE', #18028, #10754, #16350 ) ;
#3637=ORIENTED_EDGE ( 'NONE', *, *, #8976, .T. ) ;
#3640=DIRECTION ( 'NONE',  ( -7.087422195345011518E-32, -1.000000000000000000, -0.000000000000000000 ) ) ;
#3642=DIRECTION ( 'NONE',  ( 0.000000000000000000, 0.000000000000000000, 1.000000000000000000 ) ) ;
#3647=ADVANCED_FACE ( 'NONE', ( #18317 ), #3693, .T. ) ;
#3654=CARTESIAN_POINT ( 'NONE',  ( -2.413812496766188698, -9.000000000000003553, 5.000000000000079936 ) ) ;
#3661=DIRECTION ( 'NONE',  ( 0.000000000000000000, 0.000000000000000000, 1.000000000000000000 ) ) ;
#3664=EDGE_CURVE ( 'NONE', #4715, #21630, #9242, .T. ) ;
#3665=ORIENTED_EDGE ( 'NONE', *, *, #9394, .T. ) ;
#3668=ORIENTED_EDGE ( 'NONE', *, *, #18149, .T. ) ;
#3669=CARTESIAN_POINT ( 'NONE',  ( -5.564649990716551642, -8.974600000000002353, 5.000000000000079936 ) ) ;
#3670=VERTEX_POINT ( 'NONE', #16761 ) ;
#3676=ORIENTED_EDGE ( 'NONE', *, *, #13932, .F. ) ;
#3681=FACE_OUTER_BOUND ( 'NONE', #5611, .T. ) ;
#3683=CARTESIAN_POINT ( 'NONE',  ( 45.00000000000000000, 10.00000000000001599, 34.11836509645781490 ) ) ;
#3693=PLANE ( 'NONE',  #8269 ) ;
#3694=ORIENTED_EDGE ( 'NONE', *, *, #5667, .T. ) ;
#3695=DIRECTION ( 'NONE',  ( -0.3420201433256622181, 0.9396926207859106484, 1.232595164407828100E-31 ) ) ;
#3696=ORIENTED_EDGE ( 'NONE', *, *, #524, .T. ) ;
#3701=DIRECTION ( 'NONE',  ( -0.3420201433256622181, 0.9396926207859106484, 1.232595164407828100E-31 ) ) ;
#3706=DIRECTION ( 'NONE',  ( 0.000000000000000000, 0.000000000000000000, 1.000000000000000000 ) ) ;
#3710=DIRECTION ( 'NONE',  ( 0.000000000000000000, 0.000000000000000000, 1.000000000000000000 ) ) ;
#3712=CARTESIAN_POINT ( 'NONE',  ( 43.27628836966725601, -11.25000000000000355, 10.00000000000008882 ) ) ;
#3742=CARTESIAN_POINT ( 'NONE',  ( 37.81203609676620658, -9.000000000000005329, 10.00000000000008882 ) ) ;
#3761=CARTESIAN_POINT ( 'NONE',  ( 18.97172504071656363, -8.974600000000002353, 10.00000000000008882 ) ) ;
#3767=DIRECTION ( 'NONE',  ( 0.000000000000000000, 5.754033390038004481E-16, -1.000000000000000000 ) ) ;
#3773=FACE_OUTER_BOUND ( 'NONE', #22154, .T. ) ;
#3777=AXIS2_PLACEMENT_3D ( 'NONE', #2933, #4630, #8587 ) ;
#3778=DIRECTION ( 'NONE',  ( 0.3420201433256622736, 0.9396926207859106484, 0.000000000000000000 ) ) ;
#3779=DIRECTION ( 'NONE',  ( 7.087422195345011518E-32, 1.000000000000000000, -0.000000000000000000 ) ) ;
#3781=ORIENTED_EDGE ( 'NONE', *, *, #2914, .F. ) ;
#3801=VERTEX_POINT ( 'NONE', #1045 ) ;
#3807=FACE_OUTER_BOUND ( 'NONE', #18821, .T. ) ;
#3817=FILL_AREA_STYLE_COLOUR ( '', #405 ) ;
#3820=FACE_OUTER_BOUND ( 'NONE', #18493, .T. ) ;
#3821=DIRECTION ( 'NONE',  ( 7.087422195345011518E-32, 1.000000000000000000, -0.000000000000000000 ) ) ;
#3823=ORIENTED_EDGE ( 'NONE', *, *, #19180, .T. ) ;
#3825=VERTEX_POINT ( 'NONE', #20805 ) ;
#3827=EDGE_CURVE ( 'NONE', #6742, #10547, #2837, .T. ) ;
#3832=EDGE_CURVE ( 'NONE', #6714, #19393, #6216, .T. ) ;
#3837=CARTESIAN_POINT ( 'NONE',  ( -11.83859044676619199, -9.000000000000003553, 5.000000000000079936 ) ) ;
#3838=VECTOR ( 'NONE', #16086, 1000.000000000000000 ) ;
#3845=DIRECTION ( 'NONE',  ( 0.3420201433256622736, -0.9396926207859106484, -1.232595164407828100E-31 ) ) ;
#3848=VERTEX_POINT ( 'NONE', #13652 ) ;
#3850=VERTEX_POINT ( 'NONE', #10066 ) ;
#3854=LINE ( 'NONE', #9382, #963 ) ;
#3879=ORIENTED_EDGE ( 'NONE', *, *, #14404, .F. ) ;
#3883=ORIENTED_EDGE ( 'NONE', *, *, #14071, .F. ) ;
#3887=CARTESIAN_POINT ( 'NONE',  ( 50.00000000000000000, 2.399706452296377357, 55.00000000000021316 ) ) ;
#3892=CARTESIAN_POINT ( 'NONE',  ( 35.27605445928345063, -8.974600000000002353, 5.000000000000079936 ) ) ;
#3897=CARTESIAN_POINT ( 'NONE',  ( 45.00000000000000000, 15.00000000000003375, 34.11836509645780069 ) ) ;
#3899=CARTESIAN_POINT ( 'NONE',  ( 24.42673246966726452, -11.25000000000000355, 10.00000000000008882 ) ) ;
#3900=FACE_OUTER_BOUND ( 'NONE', #3340, .T. ) ;
#3905=VERTEX_POINT ( 'NONE', #16033 ) ;
#3920=CARTESIAN_POINT ( 'NONE',  ( -19.99999999999999645, -9.000000000000003553, 5.000000000000079936 ) ) ;
#3923=CARTESIAN_POINT ( 'NONE',  ( 44.00000000000000711, -9.000000000000003553, 11.00000000000008882 ) ) ;
#3933=EDGE_CURVE ( 'NONE', #6742, #12252, #14248, .T. ) ;
#3949=CARTESIAN_POINT ( 'NONE',  ( 45.00000000000000000, -15.00000000000001954, 10.00000000000008882 ) ) ;
#3955=PLANE ( 'NONE',  #19685 ) ;
#3959=DIRECTION ( 'NONE',  ( -7.087422195345011518E-32, -1.000000000000000000, -0.000000000000000000 ) ) ;
#3973=ORIENTED_EDGE ( 'NONE', *, *, #10277, .T. ) ;
#3986=VECTOR ( 'NONE', #15626, 1000.000000000000000 ) ;
#3989=CARTESIAN_POINT ( 'NONE',  ( 11.86036186966726191, -11.25000000000000355, 5.000000000000079936 ) ) ;
#3994=VECTOR ( 'NONE', #13641, 1000.000000000000000 ) ;
#3996=CARTESIAN_POINT ( 'NONE',  ( 50.00000000000000000, 7.098169556225943033, 56.71010071662853136 ) ) ;
#4003=DIRECTION ( 'NONE',  ( 0.3420201433256622736, 0.9396926207859106484, 0.000000000000000000 ) ) ;
#4018=DIRECTION ( 'NONE',  ( 0.000000000000000000, 0.000000000000000000, 1.000000000000000000 ) ) ;
#4020=CARTESIAN_POINT ( 'NONE',  ( 3.254516946766202512, -9.000000000000001776, 5.000000000000079936 ) ) ;
#4021=CARTESIAN_POINT ( 'NONE',  ( -19.99999999999999645, -9.000000000000003553, 5.000000000000079936 ) ) ;
#4029=EDGE_LOOP ( 'NONE', ( #10625, #13086, #18682, #9526 ) ) ;
#4034=EDGE_CURVE ( 'NONE', #19393, #4326, #5843, .T. ) ;
#4050=ORIENTED_EDGE ( 'NONE', *, *, #11223, .T. ) ;
#4052=CARTESIAN_POINT ( 'NONE',  ( 15.83013239071656741, -8.974600000000002353, 10.00000000000008882 ) ) ;
#4053=ORIENTED_EDGE ( 'NONE', *, *, #22032, .F. ) ;
#4059=CARTESIAN_POINT ( 'NONE',  ( 45.00000000000000000, 10.00000000000001599, 34.11836509645781490 ) ) ;
#4060=ORIENTED_EDGE ( 'NONE', *, *, #9816, .F. ) ;
#4064=ADVANCED_FACE ( 'NONE', ( #3681 ), #20436, .F. ) ;
#4067=CARTESIAN_POINT ( 'NONE',  ( 25.25491034071656316, -8.974600000000002353, 5.000000000000079936 ) ) ;
#4072=EDGE_CURVE ( 'NONE', #15000, #2759, #23296, .T. ) ;
#4075=CARTESIAN_POINT ( 'NONE',  ( -15.58579410928343911, -8.974600000000002353, 5.000000000000079936 ) ) ;
#4080=DIRECTION ( 'NONE',  ( 0.000000000000000000, 0.000000000000000000, -1.000000000000000000 ) ) ;
#4090=ORIENTED_EDGE ( 'NONE', *, *, #22819, .F. ) ;
#4095=EDGE_CURVE ( 'NONE', #1550, #1016, #18305, .T. ) ;
#4099=FACE_OUTER_BOUND ( 'NONE', #369, .T. ) ;
#4108=LINE ( 'NONE', #9286, #21410 ) ;
#4109=AXIS2_PLACEMENT_3D ( 'NONE', #11749, #2839, #8380 ) ;
#4111=DIRECTION ( 'NONE',  ( 0.3420201433256622181, -0.9396926207859107594, 0.000000000000000000 ) ) ;
#4120=CIRCLE ( 'NONE', #17887, 5.000000000000011546 ) ;
#4124=VECTOR ( 'NONE', #2433, 1000.000000000000000 ) ;
#4128=EDGE_CURVE ( 'NONE', #21720, #18422, #9230, .T. ) ;
#4138=CARTESIAN_POINT ( 'NONE',  ( 25.85127650928345489, -8.974600000000002353, 5.000000000000079936 ) ) ;
#4141=LINE ( 'NONE', #18507, #16305 ) ;
#4149=CARTESIAN_POINT ( 'NONE',  ( 50.00000000000000000, -10.00000000000001599, 34.11836509645782201 ) ) ;
#4157=ORIENTED_EDGE ( 'NONE', *, *, #8689, .F. ) ;
#4162=FACE_OUTER_BOUND ( 'NONE', #12940, .T. ) ;
#4170=AXIS2_PLACEMENT_3D ( 'NONE', #10797, #8516, #12470 ) ;
#4177=VERTEX_POINT ( 'NONE', #7659 ) ;
#4181=( GEOMETRIC_REPRESENTATION_CONTEXT ( 3 ) GLOBAL_UNCERTAINTY_ASSIGNED_CONTEXT ( ( #11724 ) ) GLOBAL_UNIT_ASSIGNED_CONTEXT ( ( #11029, #894, #3051 ) ) REPRESENTATION_CONTEXT ( 'NONE', 'WORKASPACE' ) );
#4185=CARTESIAN_POINT ( 'NONE',  ( 3.860127959283449428, -8.974600000000002353, 5.000000000000079936 ) ) ;
#4186=DIRECTION ( 'NONE',  ( -1.000000000000000000, -7.703719777548943412E-32, 0.000000000000000000 ) ) ;
#4190=AXIS2_PLACEMENT_3D ( 'NONE', #7911, #16772, #4186 ) ;
#4192=VECTOR ( 'NONE', #9666, 1000.000000000000000 ) ;
#4201=DIRECTION ( 'NONE',  ( 0.000000000000000000, 0.000000000000000000, -1.000000000000000000 ) ) ;
#4203=CARTESIAN_POINT ( 'NONE',  ( 1.546713180332750293, -11.25000000000000355, 10.00000000000008882 ) ) ;
#4213=ORIENTED_EDGE ( 'NONE', *, *, #3827, .T. ) ;
#4218=EDGE_CURVE ( 'NONE', #20787, #12158, #17467, .T. ) ;
#4225=FACE_OUTER_BOUND ( 'NONE', #847, .T. ) ;
#4232=VECTOR ( 'NONE', #23050, 1000.000000000000114 ) ;
#4233=VERTEX_POINT ( 'NONE', #11509 ) ;
#4236=ORIENTED_EDGE ( 'NONE', *, *, #17941, .F. ) ;
#4249=EDGE_CURVE ( 'NONE', #21235, #16763, #6152, .T. ) ;
#4255=LINE ( 'NONE', #11589, #15455 ) ;
#4263=VERTEX_POINT ( 'NONE', #13355 ) ;
#4274=EDGE_CURVE ( 'NONE', #7229, #9962, #17050, .T. ) ;
#4280=ORIENTED_EDGE ( 'NONE', *, *, #11223, .F. ) ;
#4284=DIRECTION ( 'NONE',  ( 1.000000000000000000, 7.703719777548943412E-32, 0.000000000000000000 ) ) ;
#4286=LINE ( 'NONE', #22471, #965 ) ;
#4290=VERTEX_POINT ( 'NONE', #11680 ) ;
#4292=DIRECTION ( 'NONE',  ( -0.000000000000000000, 0.000000000000000000, -1.000000000000000000 ) ) ;
#4293=ORIENTED_EDGE ( 'NONE', *, *, #10128, .T. ) ;
#4300=EDGE_LOOP ( 'NONE', ( #22034, #7914, #18353, #8052 ) ) ;
#4321=CARTESIAN_POINT ( 'NONE',  ( 50.38765154071656838, -8.974600000000002353, 5.000000000000079936 ) ) ;
#4326=VERTEX_POINT ( 'NONE', #13119 ) ;
#4328=ORIENTED_EDGE ( 'NONE', *, *, #21516, .F. ) ;
#4333=VECTOR ( 'NONE', #12410, 1000.000000000000000 ) ;
#4341=CARTESIAN_POINT ( 'NONE',  ( -6.161016159283438931, -8.974600000000002353, 5.000000000000079936 ) ) ;
#4345=VECTOR ( 'NONE', #14591, 1000.000000000000000 ) ;
#4356=LINE ( 'NONE', #13489, #11041 ) ;
#4364=EDGE_CURVE ( 'NONE', #22188, #9402, #20851, .T. ) ;
#4365=DIRECTION ( 'NONE',  ( 0.3420201433256622181, 0.9396926207859107594, -6.162975822039141593E-32 ) ) ;
#4372=DIRECTION ( 'NONE',  ( 0.000000000000000000, 0.000000000000000000, -1.000000000000000000 ) ) ;
#4373=CARTESIAN_POINT ( 'NONE',  ( 20.39626908033275043, -11.25000000000000355, 5.000000000000079936 ) ) ;
#4374=LINE ( 'NONE', #20321, #18115 ) ;
#4376=VERTEX_POINT ( 'NONE', #3132 ) ;
#4382=ORIENTED_EDGE ( 'NONE', *, *, #8196, .F. ) ;
#4384=CARTESIAN_POINT ( 'NONE',  ( 47.84242505928347100, -8.974600000000002353, 5.000000000000079936 ) ) ;
#4386=DIRECTION ( 'NONE',  ( 0.000000000000000000, 0.000000000000000000, -1.000000000000000000 ) ) ;
#4387=EDGE_CURVE ( 'NONE', #18254, #23165, #11920, .T. ) ;
#4389=VECTOR ( 'NONE', #9008, 1000.000000000000000 ) ;
#4402=DIRECTION ( 'NONE',  ( -7.087422195345011518E-32, -1.000000000000000000, 0.000000000000000000 ) ) ;
#4412=VECTOR ( 'NONE', #5222, 1000.000000000000000 ) ;
#4415=PLANE ( 'NONE',  #14523 ) ;
#4416=ORIENTED_EDGE ( 'NONE', *, *, #22909, .T. ) ;
#4419=DIRECTION ( 'NONE',  ( 0.3420201433256622181, -0.9396926207859107594, 0.000000000000000000 ) ) ;
#4422=DIRECTION ( 'NONE',  ( 0.000000000000000000, 0.000000000000000000, -1.000000000000000000 ) ) ;
#4425=AXIS2_PLACEMENT_3D ( 'NONE', #20389, #22306, #14933 ) ;
#4434=DIRECTION ( 'NONE',  ( 7.087422195345011518E-32, 1.000000000000000000, -0.000000000000000000 ) ) ;
#4435=ORIENTED_EDGE ( 'NONE', *, *, #15774, .F. ) ;
#4438=DIRECTION ( 'NONE',  ( -1.000000000000000000, -7.703719777548943412E-32, 0.000000000000000000 ) ) ;
#4439=LINE ( 'NONE', #6600, #11912 ) ;
#4440=ORIENTED_EDGE ( 'NONE', *, *, #17941, .T. ) ;
#4442=ORIENTED_EDGE ( 'NONE', *, *, #9095, .F. ) ;
#4445=ORIENTED_EDGE ( 'NONE', *, *, #23101, .T. ) ;
#4454=LINE ( 'NONE', #7948, #16407 ) ;
#4460=LINE ( 'NONE', #11922, #14191 ) ;
#4463=ORIENTED_EDGE ( 'NONE', *, *, #18863, .T. ) ;
#4473=VERTEX_POINT ( 'NONE', #17647 ) ;
#4483=DIRECTION ( 'NONE',  ( 1.000000000000000000, 7.703719777548943412E-32, 0.000000000000000000 ) ) ;
#4501=FACE_OUTER_BOUND ( 'NONE', #13165, .T. ) ;
#4511=ORIENTED_EDGE ( 'NONE', *, *, #4218, .T. ) ;
#4515=DIRECTION ( 'NONE',  ( 0.000000000000000000, 0.000000000000000000, -1.000000000000000000 ) ) ;
#4522=CARTESIAN_POINT ( 'NONE',  ( 47.23681404676619877, -9.000000000000003553, 5.000000000000079936 ) ) ;
#4525=LINE ( 'NONE', #8142, #13128 ) ;
#4527=CARTESIAN_POINT ( 'NONE',  ( -1.594879469667249916, -11.25000000000000355, 10.00000000000008882 ) ) ;
#4530=PRODUCT_DEFINITION_CONTEXT ( 'detailed design', #21519, 'design' ) ;
#4533=ORIENTED_EDGE ( 'NONE', *, *, #14379, .F. ) ;
#4536=DIRECTION ( 'NONE',  ( 0.000000000000000000, 0.000000000000000000, 1.000000000000000000 ) ) ;
#4554=ORIENTED_EDGE ( 'NONE', *, *, #23267, .F. ) ;
#4566=AXIS2_PLACEMENT_3D ( 'NONE', #10772, #16489, #18046 ) ;
#4569=CARTESIAN_POINT ( 'NONE',  ( 22.11331769071655984, -8.974600000000002353, 5.000000000000079936 ) ) ;
#4570=VERTEX_POINT ( 'NONE', #16433 ) ;
#4572=ORIENTED_EDGE ( 'NONE', *, *, #23437, .T. ) ;
#4575=ADVANCED_FACE ( 'NONE', ( #3368 ), #5408, .F. ) ;
#4580=CARTESIAN_POINT ( 'NONE',  ( -19.55556463033274284, -11.25000000000000355, 5.000000000000079936 ) ) ;
#4582=DIRECTION ( 'NONE',  ( 0.000000000000000000, -3.469446951953615175E-16, -1.000000000000000000 ) ) ;
#4586=CARTESIAN_POINT ( 'NONE',  ( 29.82104703033275328, -11.25000000000000355, 5.000000000000079936 ) ) ;
#4587=AXIS2_PLACEMENT_3D ( 'NONE', #968, #20731, #2417 ) ;
#4597=CARTESIAN_POINT ( 'NONE',  ( 47.24605889071655440, -8.974600000000002353, 10.00000000000008882 ) ) ;
#4607=DIRECTION ( 'NONE',  ( 0.000000000000000000, 0.000000000000000000, 1.000000000000000000 ) ) ;
#4614=CARTESIAN_POINT ( 'NONE',  ( 10.15255810323380992, -9.000000000000001776, 10.00000000000008882 ) ) ;
#4627=CARTESIAN_POINT ( 'NONE',  ( 34.36634005239895373, 10.78772952506732175, 10.00000000000008882 ) ) ;
#4630=DIRECTION ( 'NONE',  ( -7.087422195345011518E-32, -1.000000000000000000, -0.000000000000000000 ) ) ;
#4634=VERTEX_POINT ( 'NONE', #3712 ) ;
#4648=CARTESIAN_POINT ( 'NONE',  ( 5.577176569667260608, -11.25000000000000355, 5.000000000000079936 ) ) ;
#4673=ADVANCED_FACE ( 'NONE', ( #1441 ), #23371, .F. ) ;
#4675=ORIENTED_EDGE ( 'NONE', *, *, #22199, .F. ) ;
#4683=ORIENTED_EDGE ( 'NONE', *, *, #6472, .F. ) ;
#4686=LINE ( 'NONE', #15737, #13296 ) ;
#4701=ADVANCED_FACE ( 'NONE', ( #16548 ), #11656, .F. ) ;
#4715=VERTEX_POINT ( 'NONE', #5768 ) ;
#4733=EDGE_CURVE ( 'NONE', #13757, #2729, #15243, .T. ) ;
#4738=CARTESIAN_POINT ( 'NONE',  ( 25.86052135323381407, -9.000000000000001776, 10.00000000000008882 ) ) ;
#4740=ORIENTED_EDGE ( 'NONE', *, *, #11011, .T. ) ;
#4741=ORIENTED_EDGE ( 'NONE', *, *, #14745, .T. ) ;
#4754=DIRECTION ( 'NONE',  ( -1.000000000000000000, -7.703719777548943412E-32, 0.000000000000000000 ) ) ;
#4766=ORIENTED_EDGE ( 'NONE', *, *, #20431, .T. ) ;
#4775=ORIENTED_EDGE ( 'NONE', *, *, #8623, .T. ) ;
#4789=LINE ( 'NONE', #1298, #23520 ) ;
#4790=ORIENTED_EDGE ( 'NONE', *, *, #7529, .T. ) ;
#4796=EDGE_CURVE ( 'NONE', #16763, #12570, #487, .T. ) ;
#4797=EDGE_CURVE ( 'NONE', #5511, #5170, #13325, .T. ) ;
#4803=LINE ( 'NONE', #10107, #13346 ) ;
#4808=AXIS2_PLACEMENT_3D ( 'NONE', #6362, #22750, #13677 ) ;
#4842=LINE ( 'NONE', #15657, #13015 ) ;
#4844=VERTEX_POINT ( 'NONE', #15600 ) ;
#4864=EDGE_CURVE ( 'NONE', #18254, #19389, #22868, .T. ) ;
#4872=VECTOR ( 'NONE', #13723, 1000.000000000000000 ) ;
#4873=CARTESIAN_POINT ( 'NONE',  ( 118.3095189484530181, -10.00000000000001954, 15.00000000000002842 ) ) ;
#4879=VECTOR ( 'NONE', #576, 1000.000000000000114 ) ;
#4881=CARTESIAN_POINT ( 'NONE',  ( 45.52901028033275566, -11.25000000000000355, 5.000000000000079936 ) ) ;
#4886=ORIENTED_EDGE ( 'NONE', *, *, #7529, .F. ) ;
#4896=ORIENTED_EDGE ( 'NONE', *, *, #12326, .F. ) ;
#4907=CARTESIAN_POINT ( 'NONE',  ( -19.99999999999999645, -15.00000000000001954, 5.000000000000079936 ) ) ;
#4908=CARTESIAN_POINT ( 'NONE',  ( -11.84783529071655295, -8.974600000000002353, 5.000000000000079936 ) ) ;
#4909=CARTESIAN_POINT ( 'NONE',  ( 9.537702246766203373, -9.000000000000003553, 5.000000000000079936 ) ) ;
#4917=ORIENTED_EDGE ( 'NONE', *, *, #4364, .T. ) ;
#4918=VECTOR ( 'NONE', #8120, 1000.000000000000114 ) ;
#4921=DIRECTION ( 'NONE',  ( 0.000000000000000000, 0.000000000000000000, -1.000000000000000000 ) ) ;
#4924=AXIS2_PLACEMENT_3D ( 'NONE', #18831, #5660, #9169 ) ;
#4930=EDGE_CURVE ( 'NONE', #23288, #2408, #1186, .T. ) ;
#4937=ORIENTED_EDGE ( 'NONE', *, *, #22701, .F. ) ;
#4944=EDGE_CURVE ( 'NONE', #3850, #17912, #8522, .T. ) ;
#4961=VECTOR ( 'NONE', #2265, 1000.000000000000114 ) ;
#4962=LINE ( 'NONE', #14077, #8555 ) ;
#4974=CARTESIAN_POINT ( 'NONE',  ( 12.68853974071656232, -8.974600000000002353, 5.000000000000079936 ) ) ;
#4979=ADVANCED_FACE ( 'NONE', ( #15480 ), #21060, .T. ) ;
#4980=VERTEX_POINT ( 'NONE', #19271 ) ;
#4982=CARTESIAN_POINT ( 'NONE',  ( 15.00195451966726523, -11.25000000000000355, 5.000000000000079936 ) ) ;
#4999=CARTESIAN_POINT ( 'NONE',  ( 30.70991776966726405, -11.25000000000000355, 5.000000000000079936 ) ) ;
#5000=CARTESIAN_POINT ( 'NONE',  ( 17.25467643033275067, -11.25000000000000355, 5.000000000000079936 ) ) ;
#5001=ORIENTED_EDGE ( 'NONE', *, *, #14664, .F. ) ;
#5005=VECTOR ( 'NONE', #19399, 1000.000000000000114 ) ;
#5008=DIRECTION ( 'NONE',  ( 0.000000000000000000, 0.000000000000000000, 1.000000000000000000 ) ) ;
#5011=ORIENTED_EDGE ( 'NONE', *, *, #14342, .F. ) ;
#5017=DIRECTION ( 'NONE',  ( 0.000000000000000000, 0.000000000000000000, -1.000000000000000000 ) ) ;
#5020=AXIS2_PLACEMENT_3D ( 'NONE', #15365, #4434, #6236 ) ;
#5025=CARTESIAN_POINT ( 'NONE',  ( 49.55947366966726264, -11.25000000000000355, 10.00000000000008882 ) ) ;
#5031=EDGE_CURVE ( 'NONE', #1981, #22779, #22116, .T. ) ;
#5037=DIRECTION ( 'NONE',  ( 0.000000000000000000, 0.000000000000000000, 1.000000000000000000 ) ) ;
#5052=PLANE ( 'NONE',  #14575 ) ;
#5060=ORIENTED_EDGE ( 'NONE', *, *, #4249, .T. ) ;
#5062=ORIENTED_EDGE ( 'NONE', *, *, #9563, .F. ) ;
#5073=EDGE_CURVE ( 'NONE', #22188, #16559, #22608, .T. ) ;
#5078=CARTESIAN_POINT ( 'NONE',  ( 30.70991776966726405, -11.25000000000000355, 10.00000000000008882 ) ) ;
#5085=CARTESIAN_POINT ( 'NONE',  ( -5.555405146766188906, -9.000000000000003553, 5.000000000000079936 ) ) ;
#5086=ORIENTED_EDGE ( 'NONE', *, *, #12623, .T. ) ;
#5087=ORIENTED_EDGE ( 'NONE', *, *, #3832, .T. ) ;
#5089=DIRECTION ( 'NONE',  ( 0.000000000000000000, 0.000000000000000000, 1.000000000000000000 ) ) ;
#5090=ORIENTED_EDGE ( 'NONE', *, *, #6410, .F. ) ;
#5091=DIRECTION ( 'NONE',  ( 0.3420201433256622181, 0.9396926207859107594, -6.162975822039141593E-32 ) ) ;
#5095=ADVANCED_FACE ( 'NONE', ( #2598 ), #22478, .F. ) ;
#5096=ORIENTED_EDGE ( 'NONE', *, *, #21430, .F. ) ;
#5097=FACE_OUTER_BOUND ( 'NONE', #163, .T. ) ;
#5108=CARTESIAN_POINT ( 'NONE',  ( 40.13469571966727045, -11.25000000000000355, 5.000000000000079936 ) ) ;
#5118=CARTESIAN_POINT ( 'NONE',  ( 50.00000000000000000, 15.00000000000004263, 34.11836509645781490 ) ) ;
#5119=ORIENTED_EDGE ( 'NONE', *, *, #10428, .T. ) ;
#5125=FACE_OUTER_BOUND ( 'NONE', #16038, .T. ) ;
#5129=ADVANCED_FACE ( 'NONE', ( #8018 ), #21030, .F. ) ;
#5138=ORIENTED_EDGE ( 'NONE', *, *, #27, .T. ) ;
#5147=VERTEX_POINT ( 'NONE', #918 ) ;
#5149=VERTEX_POINT ( 'NONE', #6332 ) ;
#5150=LINE ( 'NONE', #8890, #7206 ) ;
#5157=VECTOR ( 'NONE', #19980, 1000.000000000000000 ) ;
#5159=AXIS2_PLACEMENT_3D ( 'NONE', #1777, #5262, #11031 ) ;
#5168=CARTESIAN_POINT ( 'NONE',  ( -19.99999999999999645, -9.000000000000003553, 5.000000000000079936 ) ) ;
#5170=VERTEX_POINT ( 'NONE', #15574 ) ;
#5175=DIRECTION ( 'NONE',  ( 0.000000000000000000, 0.000000000000000000, 1.000000000000000000 ) ) ;
#5177=CARTESIAN_POINT ( 'NONE',  ( 6.405354440716562792, -8.974600000000002353, 5.000000000000079936 ) ) ;
#5178=AXIS2_PLACEMENT_3D ( 'NONE', #17907, #7135, #1484 ) ;
#5179=ORIENTED_EDGE ( 'NONE', *, *, #18587, .F. ) ;
#5184=DIRECTION ( 'NONE',  ( -7.087422195345011518E-32, -1.000000000000000000, -0.000000000000000000 ) ) ;
#5198=VERTEX_POINT ( 'NONE', #6087 ) ;
#5210=LINE ( 'NONE', #15892, #14098 ) ;
#5216=CARTESIAN_POINT ( 'NONE',  ( -19.55556463033274284, -11.25000000000000355, 5.000000000000079936 ) ) ;
#5222=DIRECTION ( 'NONE',  ( 0.000000000000000000, 0.000000000000000000, 1.000000000000000000 ) ) ;
#5223=EDGE_CURVE ( 'NONE', #1016, #16967, #15690, .T. ) ;
#5231=LINE ( 'NONE', #17934, #8332 ) ;
#5236=ORIENTED_EDGE ( 'NONE', *, *, #21069, .T. ) ;
#5243=PLANE ( 'NONE',  #5691 ) ;
#5244=ORIENTED_EDGE ( 'NONE', *, *, #22032, .T. ) ;
#5252=DIRECTION ( 'NONE',  ( -0.3420201433256622181, 0.9396926207859106484, 1.232595164407828100E-31 ) ) ;
#5255=CARTESIAN_POINT ( 'NONE',  ( 44.00000000000000711, -9.000000000000003553, 11.00000000000008882 ) ) ;
#5261=ORIENTED_EDGE ( 'NONE', *, *, #18561, .F. ) ;
#5262=DIRECTION ( 'NONE',  ( 7.087422195345011518E-32, 1.000000000000000000, -0.000000000000000000 ) ) ;
#5270=ADVANCED_FACE ( 'NONE', ( #23317 ), #12696, .F. ) ;
#5280=DIRECTION ( 'NONE',  ( 0.000000000000000000, 0.000000000000000000, -1.000000000000000000 ) ) ;
#5292=VECTOR ( 'NONE', #18609, 1000.000000000000000 ) ;
#5318=LINE ( 'NONE', #3520, #17966 ) ;
#5321=FACE_OUTER_BOUND ( 'NONE', #604, .T. ) ;
#5332=DIRECTION ( 'NONE',  ( -7.087422195345011518E-32, -1.000000000000000000, -0.000000000000000000 ) ) ;
#5333=COLOUR_RGB ( '', 0.66274510, 0.83137255, 0.94901961) ;
#5343=PLANE ( 'NONE',  #1118 ) ;
#5348=CARTESIAN_POINT ( 'NONE',  ( -19.99999999999999645, -9.000000000000003553, 5.000000000000079936 ) ) ;
#5349=CARTESIAN_POINT ( 'NONE',  ( 50.00000000000000000, -7.098169556225942145, 56.71010071662853136 ) ) ;
#5353=CARTESIAN_POINT ( 'NONE',  ( 50.00000000000000711, -10.03966385473555789, 5.000000000000079936 ) ) ;
#5356=EDGE_LOOP ( 'NONE', ( #12306, #7138, #18058, #20002 ) ) ;
#5357=VECTOR ( 'NONE', #22801, 1000.000000000000000 ) ;
#5372=CARTESIAN_POINT ( 'NONE',  ( 30.70991776966726405, -11.25000000000000355, 5.000000000000079936 ) ) ;
#5381=ORIENTED_EDGE ( 'NONE', *, *, #18595, .T. ) ;
#5386=ORIENTED_EDGE ( 'NONE', *, *, #15305, .T. ) ;
#5397=EDGE_CURVE ( 'NONE', #12965, #4570, #1629, .T. ) ;
#5408=PLANE ( 'NONE',  #19136 ) ;
#5411=EDGE_LOOP ( 'NONE', ( #22059, #11337, #6010, #243 ) ) ;
#5419=EDGE_CURVE ( 'NONE', #22275, #16998, #4141, .T. ) ;
#5425=ADVANCED_FACE ( 'NONE', ( #5821 ), #1859, .F. ) ;
#5447=CARTESIAN_POINT ( 'NONE',  ( -7.245101763170664455, -4.357596700699738257, 10.00000000000008882 ) ) ;
#5461=SURFACE_SIDE_STYLE ('',( #3306 ) ) ;
#5467=CYLINDRICAL_SURFACE ( 'NONE', #173, 5.000000000000011546 ) ;
#5468=ORIENTED_EDGE ( 'NONE', *, *, #23541, .T. ) ;
#5472=ORIENTED_EDGE ( 'NONE', *, *, #4944, .T. ) ;
#5477=AXIS2_PLACEMENT_3D ( 'NONE', #17290, #4582, #11795 ) ;
#5480=CARTESIAN_POINT ( 'NONE',  ( 41.56848460323381289, -9.000000000000001776, 10.00000000000008882 ) ) ;
#5481=CARTESIAN_POINT ( 'NONE',  ( -19.99999999999999645, -9.000000000000003553, 5.000000000000079936 ) ) ;
#5485=LINE ( 'NONE', #16283, #16803 ) ;
#5488=DIRECTION ( 'NONE',  ( 0.000000000000000000, 0.000000000000000000, -1.000000000000000000 ) ) ;
#5492=VERTEX_POINT ( 'NONE', #7288 ) ;
#5493=LINE ( 'NONE', #12721, #10105 ) ;
#5509=DIRECTION ( 'NONE',  ( 1.000000000000000000, 7.703719777548943412E-32, 0.000000000000000000 ) ) ;
#5511=VERTEX_POINT ( 'NONE', #70 ) ;
#5523=EDGE_CURVE ( 'NONE', #7050, #22527, #16607, .T. ) ;
#5529=EDGE_CURVE ( 'NONE', #2345, #19331, #20174, .T. ) ;
#5557=EDGE_CURVE ( 'NONE', #21366, #9385, #14960, .T. ) ;
#5574=CARTESIAN_POINT ( 'NONE',  ( -19.99999999999999645, -9.000000000000003553, 5.000000000000079936 ) ) ;
#5579=AXIS2_PLACEMENT_3D ( 'NONE', #17109, #10181, #1155 ) ;
#5580=LINE ( 'NONE', #11230, #1352 ) ;
#5585=EDGE_CURVE ( 'NONE', #19783, #12772, #1014, .T. ) ;
#5595=ORIENTED_EDGE ( 'NONE', *, *, #23008, .F. ) ;
#5611=EDGE_LOOP ( 'NONE', ( #16531, #9922, #21319, #7484 ) ) ;
#5614=CARTESIAN_POINT ( 'NONE',  ( 18.96248019676620444, -9.000000000000005329, 10.00000000000008882 ) ) ;
#5616=LINE ( 'NONE', #13650, #19307 ) ;
#5619=ADVANCED_FACE ( 'NONE', ( #14515 ), #21779, .F. ) ;
#5620=ORIENTED_EDGE ( 'NONE', *, *, #19578, .T. ) ;
#5627=DIRECTION ( 'NONE',  ( 0.000000000000000000, 0.000000000000000000, -1.000000000000000000 ) ) ;
#5632=VECTOR ( 'NONE', #9594, 1000.000000000000000 ) ;
#5637=FACE_OUTER_BOUND ( 'NONE', #2927, .T. ) ;
#5649=ORIENTED_EDGE ( 'NONE', *, *, #4218, .F. ) ;
#5660=DIRECTION ( 'NONE',  ( 0.000000000000000000, -0.000000000000000000, 1.000000000000000000 ) ) ;
#5667=EDGE_CURVE ( 'NONE', #18990, #2345, #7326, .T. ) ;
#5676=EDGE_LOOP ( 'NONE', ( #5776, #18021, #10213, #20303 ) ) ;
#5683=LINE ( 'NONE', #13019, #17112 ) ;
#5691=AXIS2_PLACEMENT_3D ( 'NONE', #12587, #7306, #23334 ) ;
#5692=LINE ( 'NONE', #13027, #4192 ) ;
#5696=EDGE_CURVE ( 'NONE', #15755, #3801, #18540, .T. ) ;
#5700=LINE ( 'NONE', #20171, #12099 ) ;
#5701=ORIENTED_EDGE ( 'NONE', *, *, #21731, .T. ) ;
#5704=DIRECTION ( 'NONE',  ( 0.000000000000000000, 0.000000000000000000, 1.000000000000000000 ) ) ;
#5705=CARTESIAN_POINT ( 'NONE',  ( -19.99999999999999645, -9.000000000000003553, 10.00000000000008882 ) ) ;
#5711=VERTEX_POINT ( 'NONE', #11267 ) ;
#5738=CARTESIAN_POINT ( 'NONE',  ( -19.99999999999999645, -9.000000000000003553, 10.00000000000008882 ) ) ;
#5745=CARTESIAN_POINT ( 'NONE',  ( 38.41764710928345750, -8.974600000000002353, 5.000000000000079936 ) ) ;
#5746=VERTEX_POINT ( 'NONE', #7546 ) ;
#5749=CYLINDRICAL_SURFACE ( 'NONE', #17920, 2.500000000000009326 ) ;
#5765=EDGE_CURVE ( 'NONE', #11172, #11370, #16527, .T. ) ;
#5768=CARTESIAN_POINT ( 'NONE',  ( 13.29415075323381323, -9.000000000000001776, 10.00000000000008882 ) ) ;
#5776=ORIENTED_EDGE ( 'NONE', *, *, #19878, .T. ) ;
#5794=ORIENTED_EDGE ( 'NONE', *, *, #22940, .T. ) ;
#5801=CARTESIAN_POINT ( 'NONE',  ( 7.010965453233809264, -9.000000000000001776, 10.00000000000008882 ) ) ;
#5804=ADVANCED_FACE ( 'NONE', ( #2128 ), #9463, .T. ) ;
#5806=LINE ( 'NONE', #20751, #16378 ) ;
#5807=ORIENTED_EDGE ( 'NONE', *, *, #17642, .F. ) ;
#5817=CARTESIAN_POINT ( 'NONE',  ( 45.00000000000000000, 10.00000000000001599, 34.11836509645781490 ) ) ;
#5819=ORIENTED_EDGE ( 'NONE', *, *, #17341, .F. ) ;
#5821=FACE_OUTER_BOUND ( 'NONE', #12451, .T. ) ;
#5825=EDGE_CURVE ( 'NONE', #3670, #12921, #102, .T. ) ;
#5831=ORIENTED_EDGE ( 'NONE', *, *, #9670, .T. ) ;
#5838=VERTEX_POINT ( 'NONE', #10065 ) ;
#5843=LINE ( 'NONE', #18187, #11078 ) ;
#5844=CARTESIAN_POINT ( 'NONE',  ( 43.27628836966725601, -11.25000000000000355, 10.00000000000008882 ) ) ;
#5845=DIRECTION ( 'NONE',  ( 1.000000000000000000, 7.703719777548943412E-32, 0.000000000000000000 ) ) ;
#5847=ORIENTED_EDGE ( 'NONE', *, *, #20642, .T. ) ;
#5850=EDGE_CURVE ( 'NONE', #6494, #22779, #11746, .T. ) ;
#5852=FILL_AREA_STYLE ('',( #3817 ) ) ;
#5855=DIRECTION ( 'NONE',  ( 0.000000000000000000, 0.000000000000000000, 1.000000000000000000 ) ) ;
#5858=EDGE_CURVE ( 'NONE', #17335, #6815, #9821, .T. ) ;
#5866=DIRECTION ( 'NONE',  ( 0.3420201433256622736, -0.9396926207859106484, -1.232595164407828100E-31 ) ) ;
#5886=ORIENTED_EDGE ( 'NONE', *, *, #11859, .F. ) ;
#5894=PLANE ( 'NONE',  #16654 ) ;
#5895=ORIENTED_EDGE ( 'NONE', *, *, #10123, .T. ) ;
#5899=EDGE_CURVE ( 'NONE', #19009, #12570, #13890, .T. ) ;
#5924=VECTOR ( 'NONE', #8746, 1000.000000000000000 ) ;
#5931=ADVANCED_FACE ( 'NONE', ( #15694 ), #813, .F. ) ;
#5932=VECTOR ( 'NONE', #7325, 1000.000000000000114 ) ;
#5933=DIRECTION ( 'NONE',  ( 0.000000000000000000, 0.000000000000000000, -1.000000000000000000 ) ) ;
#5945=ORIENTED_EDGE ( 'NONE', *, *, #21430, .T. ) ;
#5968=FACE_OUTER_BOUND ( 'NONE', #22405, .T. ) ;
#5979=FACE_BOUND ( 'NONE', #21559, .T. ) ;
#5983=CARTESIAN_POINT ( 'NONE',  ( 28.81814781032300488, 8.768352694965047434, 10.00000000000008882 ) ) ;
#5986=FACE_OUTER_BOUND ( 'NONE', #11546, .T. ) ;
#6000=DIRECTION ( 'NONE',  ( 0.3420201433256622181, 0.9396926207859107594, -6.162975822039141593E-32 ) ) ;
#6001=EDGE_CURVE ( 'NONE', #7167, #6956, #7294, .T. ) ;
#6010=ORIENTED_EDGE ( 'NONE', *, *, #13216, .F. ) ;
#6016=VECTOR ( 'NONE', #1370, 1000.000000000000000 ) ;
#6032=ORIENTED_EDGE ( 'NONE', *, *, #16551, .F. ) ;
#6034=ORIENTED_EDGE ( 'NONE', *, *, #10964, .T. ) ;
#6043=VECTOR ( 'NONE', #10899, 1000.000000000000000 ) ;
#6058=LINE ( 'NONE', #11115, #18959 ) ;
#6065=VECTOR ( 'NONE', #21147, 1000.000000000000000 ) ;
#6067=CARTESIAN_POINT ( 'NONE',  ( 38.42689195323381313, -9.000000000000001776, 5.000000000000079936 ) ) ;
#6072=AXIS2_PLACEMENT_3D ( 'NONE', #12052, #14315, #15872 ) ;
#6074=VERTEX_POINT ( 'NONE', #8725 ) ;
#6075=PLANE ( 'NONE',  #22466 ) ;
#6080=CARTESIAN_POINT ( 'NONE',  ( 20.49585944720908870, 5.739287449811636854, 10.00000000000008882 ) ) ;
#6082=DIRECTION ( 'NONE',  ( 0.000000000000000000, 0.000000000000000000, -1.000000000000000000 ) ) ;
#6087=CARTESIAN_POINT ( 'NONE',  ( 40.95362874676621345, -9.000000000000005329, 10.00000000000008882 ) ) ;
#6088=CARTESIAN_POINT ( 'NONE',  ( -3.847601380332740018, -11.25000000000000355, 10.00000000000008882 ) ) ;
#6098=ORIENTED_EDGE ( 'NONE', *, *, #15236, .F. ) ;
#6100=EDGE_CURVE ( 'NONE', #17999, #1835, #10888, .T. ) ;
#6104=DIRECTION ( 'NONE',  ( -7.087422195345011518E-32, -1.000000000000000000, -0.000000000000000000 ) ) ;
#6105=ORIENTED_EDGE ( 'NONE', *, *, #22819, .T. ) ;
#6112=VECTOR ( 'NONE', #11849, 1000.000000000000000 ) ;
#6117=PLANE ( 'NONE',  #931 ) ;
#6121=CARTESIAN_POINT ( 'NONE',  ( -19.99999999999999645, -9.000000000000003553, 10.00000000000008882 ) ) ;
#6127=VERTEX_POINT ( 'NONE', #12337 ) ;
#6133=CARTESIAN_POINT ( 'NONE',  ( 44.10446624071656174, -8.974600000000002353, 10.00000000000008882 ) ) ;
#6139=ORIENTED_EDGE ( 'NONE', *, *, #174, .F. ) ;
#6142=VECTOR ( 'NONE', #16606, 1000.000000000000114 ) ;
#6152=LINE ( 'NONE', #394, #13198 ) ;
#6156=ORIENTED_EDGE ( 'NONE', *, *, #13669, .T. ) ;
#6171=EDGE_CURVE ( 'NONE', #1126, #6074, #5231, .T. ) ;
#6173=VECTOR ( 'NONE', #16627, 1000.000000000000000 ) ;
#6183=DIRECTION ( 'NONE',  ( -7.087422195345011518E-32, -1.000000000000000000, -0.000000000000000000 ) ) ;
#6186=EDGE_LOOP ( 'NONE', ( #6139, #23582, #17119, #9460, #19176, #1721, #22587 ) ) ;
#6203=DIRECTION ( 'NONE',  ( -1.000000000000000000, -7.703719777548943412E-32, 0.000000000000000000 ) ) ;
#6209=ORIENTED_EDGE ( 'NONE', *, *, #12561, .T. ) ;
#6213=EDGE_LOOP ( 'NONE', ( #7351, #18786, #14606, #6611 ) ) ;
#6216=LINE ( 'NONE', #22725, #13254 ) ;
#6218=CARTESIAN_POINT ( 'NONE',  ( 40.96287359071656908, -8.974600000000002353, 10.00000000000008882 ) ) ;
#6236=DIRECTION ( 'NONE',  ( 0.000000000000000000, 0.000000000000000000, 1.000000000000000000 ) ) ;
#6237=ORIENTED_EDGE ( 'NONE', *, *, #14071, .T. ) ;
#6254=AXIS2_PLACEMENT_3D ( 'NONE', #3923, #19105, #13619 ) ;
#6262=CARTESIAN_POINT ( 'NONE',  ( 45.00000000000000000, 10.00000000000001599, 17.50000000000003197 ) ) ;
#6270=AXIS2_PLACEMENT_3D ( 'NONE', #7624, #18617, #2206 ) ;
#6271=ORIENTED_EDGE ( 'NONE', *, *, #21288, .F. ) ;
#6272=PLANE ( 'NONE',  #21188 ) ;
#6283=CARTESIAN_POINT ( 'NONE',  ( -6.161016159283438931, -8.974600000000002353, 5.000000000000079936 ) ) ;
#6287=LINE ( 'NONE', #20869, #2626 ) ;
#6308=EDGE_CURVE ( 'NONE', #4290, #14520, #18402, .T. ) ;
#6309=ORIENTED_EDGE ( 'NONE', *, *, #2197, .T. ) ;
#6313=LINE ( 'NONE', #7997, #20157 ) ;
#6315=CARTESIAN_POINT ( 'NONE',  ( 11.86036186966726191, -11.25000000000000355, 5.000000000000079936 ) ) ;
#6317=VECTOR ( 'NONE', #14477, 1000.000000000000000 ) ;
#6332=CARTESIAN_POINT ( 'NONE',  ( 29.00211400323381028, -9.000000000000005329, 5.000000000000079936 ) ) ;
#6335=ORIENTED_EDGE ( 'NONE', *, *, #6171, .T. ) ;
#6351=ORIENTED_EDGE ( 'NONE', *, *, #3664, .T. ) ;
#6352=AXIS2_PLACEMENT_3D ( 'NONE', #17632, #21179, #5037 ) ;
#6358=DIRECTION ( 'NONE',  ( -6.974779929323510821E-32, -1.000000000000000000, 5.754033390038005467E-16 ) ) ;
#6362=CARTESIAN_POINT ( 'NONE',  ( -19.99999999999999645, -9.000000000000003553, 5.000000000000079936 ) ) ;
#6367=CARTESIAN_POINT ( 'NONE',  ( 18.96248019676620444, -9.000000000000005329, 5.000000000000079936 ) ) ;
#6371=ORIENTED_EDGE ( 'NONE', *, *, #10275, .T. ) ;
#6380=LINE ( 'NONE', #13697, #19446 ) ;
#6399=ORIENTED_EDGE ( 'NONE', *, *, #6001, .T. ) ;
#6405=CARTESIAN_POINT ( 'NONE',  ( 45.00000000000000000, -15.00000000000001954, 11.00000000000008882 ) ) ;
#6407=AXIS2_PLACEMENT_3D ( 'NONE', #6671, #1251, #18039 ) ;
#6410=EDGE_CURVE ( 'NONE', #9029, #18952, #1019, .T. ) ;
#6411=DIRECTION ( 'NONE',  ( 0.000000000000000000, 0.000000000000000000, -1.000000000000000000 ) ) ;
#6426=VERTEX_POINT ( 'NONE', #2457 ) ;
#6439=EDGE_CURVE ( 'NONE', #19783, #9681, #8235, .T. ) ;
#6447=FACE_OUTER_BOUND ( 'NONE', #9497, .T. ) ;
#6452=DIRECTION ( 'NONE',  ( -1.000000000000000000, -7.703719777548943412E-32, 0.000000000000000000 ) ) ;
#6472=EDGE_CURVE ( 'NONE', #21867, #9681, #12075, .T. ) ;
#6479=PLANE ( 'NONE',  #5020 ) ;
#6487=DIRECTION ( 'NONE',  ( 0.000000000000000000, 0.000000000000000000, 1.000000000000000000 ) ) ;
#6488=VERTEX_POINT ( 'NONE', #8479 ) ;
#6492=DIRECTION ( 'NONE',  ( 1.000000000000000000, 7.703719777548943412E-32, 0.000000000000000000 ) ) ;
#6494=VERTEX_POINT ( 'NONE', #15783 ) ;
#6504=STYLED_ITEM ( 'NONE', ( #10649 ), #22288 ) ;
#6512=DIRECTION ( 'NONE',  ( 0.000000000000000000, 0.000000000000000000, 1.000000000000000000 ) ) ;
#6513=VECTOR ( 'NONE', #12026, 1000.000000000000000 ) ;
#6521=VECTOR ( 'NONE', #11858, 1000.000000000000000 ) ;
#6524=ORIENTED_EDGE ( 'NONE', *, *, #18003, .T. ) ;
#6526=ORIENTED_EDGE ( 'NONE', *, *, #7766, .F. ) ;
#6537=STYLED_ITEM ( 'NONE', ( #214 ), #449 ) ;
#6546=DIRECTION ( 'NONE',  ( 0.000000000000000000, 0.000000000000000000, -1.000000000000000000 ) ) ;
#6568=DIRECTION ( 'NONE',  ( 0.000000000000000000, 0.000000000000000000, 1.000000000000000000 ) ) ;
#6569=VERTEX_POINT ( 'NONE', #23529 ) ;
#6576=CARTESIAN_POINT ( 'NONE',  ( 2.435583919667260400, -11.25000000000000355, 5.000000000000079936 ) ) ;
#6577=ADVANCED_FACE ( 'NONE', ( #14222 ), #6667, .F. ) ;
#6581=ORIENTED_EDGE ( 'NONE', *, *, #15741, .F. ) ;
#6587=ORIENTED_EDGE ( 'NONE', *, *, #8046, .T. ) ;
#6594=CARTESIAN_POINT ( 'NONE',  ( 44.71007725323381976, -9.000000000000003553, 10.29587622221672127 ) ) ;
#6595=ORIENTED_EDGE ( 'NONE', *, *, #13517, .T. ) ;
#6600=CARTESIAN_POINT ( 'NONE',  ( 9.399474963057187438, 1.700533789607089563, 10.00000000000008882 ) ) ;
#6611=ORIENTED_EDGE ( 'NONE', *, *, #12027, .F. ) ;
#6614=CARTESIAN_POINT ( 'NONE',  ( 9.546947090716562556, -8.974600000000002353, 5.000000000000079936 ) ) ;
#6624=LINE ( 'NONE', #4586, #7678 ) ;
#6625=ORIENTED_EDGE ( 'NONE', *, *, #9262, .T. ) ;
#6626=CARTESIAN_POINT ( 'NONE',  ( -11.01965741966725076, -11.25000000000000355, 5.000000000000079936 ) ) ;
#6634=ORIENTED_EDGE ( 'NONE', *, *, #8560, .T. ) ;
#6635=DIRECTION ( 'NONE',  ( 0.3420201433256622181, 0.9396926207859107594, -6.162975822039141593E-32 ) ) ;
#6637=VECTOR ( 'NONE', #6546, 1000.000000000000000 ) ;
#6638=VECTOR ( 'NONE', #1187, 1000.000000000000000 ) ;
#6641=VERTEX_POINT ( 'NONE', #23651 ) ;
#6661=EDGE_LOOP ( 'NONE', ( #9206, #4382, #9755, #20215 ) ) ;
#6667=PLANE ( 'NONE',  #287 ) ;
#6671=CARTESIAN_POINT ( 'NONE',  ( -5.564649990716551642, -8.974600000000002353, 5.000000000000079936 ) ) ;
#6681=VERTEX_POINT ( 'NONE', #18378 ) ;
#6690=AXIS2_PLACEMENT_3D ( 'NONE', #21972, #3779, #11119 ) ;
#6694=LINE ( 'NONE', #19022, #16479 ) ;
#6710=CARTESIAN_POINT ( 'NONE',  ( -19.99999999999999645, -9.000000000000003553, 10.00000000000008882 ) ) ;
#6714=VERTEX_POINT ( 'NONE', #9534 ) ;
#6715=DIRECTION ( 'NONE',  ( 0.9396926207859107594, -0.3420201433256623291, 3.697785493223492838E-32 ) ) ;
#6718=ORIENTED_EDGE ( 'NONE', *, *, #1202, .F. ) ;
#6725=EDGE_CURVE ( 'NONE', #21534, #10010, #279, .T. ) ;
#6729=AXIS2_PLACEMENT_3D ( 'NONE', #19707, #1745, #18160 ) ;
#6732=DIRECTION ( 'NONE',  ( 1.000000000000000000, 7.703719777548943412E-32, 0.000000000000000000 ) ) ;
#6733=EDGE_CURVE ( 'NONE', #13557, #13221, #1959, .T. ) ;
#6741=CARTESIAN_POINT ( 'NONE',  ( 46.41788101966725577, -11.25000000000000355, 5.000000000000079936 ) ) ;
#6742=VERTEX_POINT ( 'NONE', #12782 ) ;
#6758=DIRECTION ( 'NONE',  ( 0.3420201433256622736, -0.9396926207859106484, -1.232595164407828100E-31 ) ) ;
#6763=EDGE_CURVE ( 'NONE', #6641, #11902, #11339, .T. ) ;
#6768=ORIENTED_EDGE ( 'NONE', *, *, #10982, .F. ) ;
#6770=DIRECTION ( 'NONE',  ( 0.000000000000000000, 0.000000000000000000, 1.000000000000000000 ) ) ;
#6771=VERTEX_POINT ( 'NONE', #2196 ) ;
#6776=EDGE_LOOP ( 'NONE', ( #6779, #15584, #2409, #22500 ) ) ;
#6779=ORIENTED_EDGE ( 'NONE', *, *, #5825, .F. ) ;
#6781=CARTESIAN_POINT ( 'NONE',  ( 50.00000000000000000, 14.69846310392956745, 35.82846581308617573 ) ) ;
#6789=LINE ( 'NONE', #14110, #13794 ) ;
#6808=VERTEX_POINT ( 'NONE', #13251 ) ;
#6812=DIRECTION ( 'NONE',  ( 0.000000000000000000, 0.000000000000000000, 1.000000000000000000 ) ) ;
#6815=VERTEX_POINT ( 'NONE', #14582 ) ;
#6827=VECTOR ( 'NONE', #14874, 1000.000000000000114 ) ;
#6829=FACE_OUTER_BOUND ( 'NONE', #8610, .T. ) ;
#6831=CARTESIAN_POINT ( 'NONE',  ( 45.00000000000000000, 2.399706452296377801, 55.00000000000021316 ) ) ;
#6837=ORIENTED_EDGE ( 'NONE', *, *, #12604, .T. ) ;
#6854=EDGE_LOOP ( 'NONE', ( #3118, #4050, #6335, #20544 ) ) ;
#6855=EDGE_CURVE ( 'NONE', #18435, #10807, #525, .T. ) ;
#6860=VECTOR ( 'NONE', #17708, 1000.000000000000114 ) ;
#6862=EDGE_CURVE ( 'NONE', #11902, #18250, #18964, .T. ) ;
#6876=LINE ( 'NONE', #23034, #18635 ) ;
#6877=DIRECTION ( 'NONE',  ( 0.000000000000000000, 0.000000000000000000, 1.000000000000000000 ) ) ;
#6887=CARTESIAN_POINT ( 'NONE',  ( 118.3095189484530181, 2.399706452296353820, 60.00000000000021316 ) ) ;
#6891=CARTESIAN_POINT ( 'NONE',  ( 45.00000000000000000, 14.69846310392956745, 35.82846581308617573 ) ) ;
#6895=VECTOR ( 'NONE', #21679, 1000.000000000000000 ) ;
#6900=ORIENTED_EDGE ( 'NONE', *, *, #21808, .F. ) ;
#6911=AXIS2_PLACEMENT_3D ( 'NONE', #22389, #3959, #11415 ) ;
#6919=DIRECTION ( 'NONE',  ( 0.000000000000000000, -0.000000000000000000, 1.000000000000000000 ) ) ;
#6923=ORIENTED_EDGE ( 'NONE', *, *, #17089, .T. ) ;
#6925=DIRECTION ( 'NONE',  ( -7.087422195345011518E-32, -1.000000000000000000, -0.000000000000000000 ) ) ;
#6926=DIRECTION ( 'NONE',  ( -0.9396926207859107594, -0.3420201433256623291, 1.540743955509804830E-32 ) ) ;
#6928=ORIENTED_EDGE ( 'NONE', *, *, #6100, .F. ) ;
#6932=VERTEX_POINT ( 'NONE', #21208 ) ;
#6941=FACE_OUTER_BOUND ( 'NONE', #21680, .T. ) ;
#6944=ORIENTED_EDGE ( 'NONE', *, *, #21808, .T. ) ;
#6951=FACE_OUTER_BOUND ( 'NONE', #1990, .T. ) ;
#6952=EDGE_LOOP ( 'NONE', ( #6900, #12222, #23531, #19688 ) ) ;
#6956=VERTEX_POINT ( 'NONE', #20977 ) ;
#6957=CARTESIAN_POINT ( 'NONE',  ( 36.99310306966726358, -11.25000000000000355, 5.000000000000079936 ) ) ;
#6974=CARTESIAN_POINT ( 'NONE',  ( 28.38725814676620018, -9.000000000000007105, 5.000000000000079936 ) ) ;
#6978=ORIENTED_EDGE ( 'NONE', *, *, #6763, .F. ) ;
#6985=ORIENTED_EDGE ( 'NONE', *, *, #8798, .F. ) ;
#6995=LINE ( 'NONE', #23146, #11844 ) ;
#7013=VECTOR ( 'NONE', #4438, 1000.000000000000000 ) ;
#7014=DIRECTION ( 'NONE',  ( 0.000000000000000000, 0.000000000000000000, 1.000000000000000000 ) ) ;
#7019=LINE ( 'NONE', #8480, #16009 ) ;
#7020=ORIENTED_EDGE ( 'NONE', *, *, #10964, .F. ) ;
#7023=EDGE_CURVE ( 'NONE', #22879, #15720, #15973, .T. ) ;
#7026=VECTOR ( 'NONE', #12477, 1000.000000000000000 ) ;
#7030=EDGE_CURVE ( 'NONE', #4263, #5746, #17765, .T. ) ;
#7046=ORIENTED_EDGE ( 'NONE', *, *, #8046, .F. ) ;
#7050=VERTEX_POINT ( 'NONE', #10484 ) ;
#7055=PLANE ( 'NONE',  #16743 ) ;
#7058=EDGE_LOOP ( 'NONE', ( #14443, #1783, #22944, #17657 ) ) ;
#7059=DIRECTION ( 'NONE',  ( 7.087422195345011518E-32, 1.000000000000000000, -0.000000000000000000 ) ) ;
#7060=EDGE_CURVE ( 'NONE', #1856, #6742, #19082, .T. ) ;
#7062=DIRECTION ( 'NONE',  ( 7.087422195345011518E-32, 1.000000000000000000, -0.000000000000000000 ) ) ;
#7067=ORIENTED_EDGE ( 'NONE', *, *, #14508, .F. ) ;
#7069=VECTOR ( 'NONE', #7777, 1000.000000000000000 ) ;
#7071=LINE ( 'NONE', #4909, #20009 ) ;
#7073=ORIENTED_EDGE ( 'NONE', *, *, #3664, .F. ) ;
#7078=VECTOR ( 'NONE', #21167, 1000.000000000000000 ) ;
#7085=LINE ( 'NONE', #14403, #9564 ) ;
#7089=AXIS2_PLACEMENT_3D ( 'NONE', #18539, #101, #7433 ) ;
#7100=DIRECTION ( 'NONE',  ( 7.087422195345011518E-32, 1.000000000000000000, -0.000000000000000000 ) ) ;
#7109=CARTESIAN_POINT ( 'NONE',  ( 19.56809120928344825, -8.974600000000002353, 5.000000000000079936 ) ) ;
#7111=ORIENTED_EDGE ( 'NONE', *, *, #15350, .T. ) ;
#7118=VECTOR ( 'NONE', #9845, 1000.000000000000114 ) ;
#7123=CARTESIAN_POINT ( 'NONE',  ( 24.42673246966726452, -11.25000000000000355, 5.000000000000079936 ) ) ;
#7124=AXIS2_PLACEMENT_3D ( 'NONE', #12368, #19631, #1194 ) ;
#7135=DIRECTION ( 'NONE',  ( -0.9396926207859107594, -0.3420201433256623291, 1.540743955509804830E-32 ) ) ;
#7138=ORIENTED_EDGE ( 'NONE', *, *, #17973, .F. ) ;
#7139=EDGE_CURVE ( 'NONE', #22026, #3850, #11159, .T. ) ;
#7142=DIRECTION ( 'NONE',  ( 0.000000000000000000, 0.000000000000000000, -1.000000000000000000 ) ) ;
#7145=CARTESIAN_POINT ( 'NONE',  ( 44.89825008461777855, -9.517000605182268202, 10.48564008399537428 ) ) ;
#7150=CARTESIAN_POINT ( 'NONE',  ( 11.86036186966726191, -11.25000000000000355, 5.000000000000079936 ) ) ;
#7156=DIRECTION ( 'NONE',  ( 0.000000000000000000, 0.000000000000000000, -1.000000000000000000 ) ) ;
#7158=ORIENTED_EDGE ( 'NONE', *, *, #441, .F. ) ;
#7159=LINE ( 'NONE', #19949, #6142 ) ;
#7167=VERTEX_POINT ( 'NONE', #16098 ) ;
#7169=ORIENTED_EDGE ( 'NONE', *, *, #18593, .F. ) ;
#7170=CARTESIAN_POINT ( 'NONE',  ( 18.14354716966726144, -11.25000000000000355, 5.000000000000079936 ) ) ;
#7171=EDGE_LOOP ( 'NONE', ( #11813, #12826, #14488, #10345 ) ) ;
#7180=CARTESIAN_POINT ( 'NONE',  ( 50.00000000000000000, 15.00000000000001954, 10.00000000000008882 ) ) ;
#7191=CARTESIAN_POINT ( 'NONE',  ( -0.7060087303327398089, -11.25000000000000355, 10.00000000000008882 ) ) ;
#7195=ADVANCED_FACE ( 'NONE', ( #21690 ), #16890, .F. ) ;
#7202=EDGE_CURVE ( 'NONE', #7460, #18054, #13186, .T. ) ;
#7205=ORIENTED_EDGE ( 'NONE', *, *, #4249, .F. ) ;
#7206=VECTOR ( 'NONE', #1307, 1000.000000000000114 ) ;
#7226=ORIENTED_EDGE ( 'NONE', *, *, #20063, .T. ) ;
#7227=VECTOR ( 'NONE', #5855, 1000.000000000000000 ) ;
#7229=VERTEX_POINT ( 'NONE', #12951 ) ;
#7235=ORIENTED_EDGE ( 'NONE', *, *, #1162, .T. ) ;
#7237=EDGE_CURVE ( 'NONE', #7712, #23556, #18432, .T. ) ;
#7240=VECTOR ( 'NONE', #9478, 1000.000000000000000 ) ;
#7243=VECTOR ( 'NONE', #19957, 1000.000000000000000 ) ;
#7260=DIRECTION ( 'NONE',  ( 0.000000000000000000, 0.000000000000000000, 1.000000000000000000 ) ) ;
#7265=VECTOR ( 'NONE', #1660, 1000.000000000000000 ) ;
#7270=CARTESIAN_POINT ( 'NONE',  ( 45.00000000000000000, -9.796556200126357083, 11.00000000000008882 ) ) ;
#7271=VECTOR ( 'NONE', #20339, 1000.000000000000000 ) ;
#7273=CIRCLE ( 'NONE', #20625, 5.000000000000011546 ) ;
#7278=DIRECTION ( 'NONE',  ( 0.000000000000000000, 0.000000000000000000, 1.000000000000000000 ) ) ;
#7288=CARTESIAN_POINT ( 'NONE',  ( 32.96263968033274949, -11.25000000000000355, 10.00000000000008882 ) ) ;
#7294=LINE ( 'NONE', #8857, #16024 ) ;
#7298=CARTESIAN_POINT ( 'NONE',  ( -19.99999999999999645, -9.000000000000003553, 5.000000000000079936 ) ) ;
#7300=VECTOR ( 'NONE', #18307, 1000.000000000000000 ) ;
#7304=DIRECTION ( 'NONE',  ( 7.087422195345010423E-32, 0.9396926207859083169, 0.3420201433256690460 ) ) ;
#7306=DIRECTION ( 'NONE',  ( -0.9396926207859107594, -0.3420201433256623291, 1.540743955509804830E-32 ) ) ;
#7311=ADVANCED_FACE ( 'NONE', ( #17880 ), #8148, .T. ) ;
#7313=LINE ( 'NONE', #327, #19538 ) ;
#7318=AXIS2_PLACEMENT_3D ( 'NONE', #3111, #10686, #17843 ) ;
#7319=ORIENTED_EDGE ( 'NONE', *, *, #27, .F. ) ;
#7323=EDGE_CURVE ( 'NONE', #18054, #14420, #17118, .T. ) ;
#7324=ORIENTED_EDGE ( 'NONE', *, *, #11048, .F. ) ;
#7325=DIRECTION ( 'NONE',  ( 0.3420201433256622181, 0.9396926207859107594, -6.162975822039141593E-32 ) ) ;
#7326=LINE ( 'NONE', #13299, #5632 ) ;
#7339=LINE ( 'NONE', #23365, #9080 ) ;
#7351=ORIENTED_EDGE ( 'NONE', *, *, #12425, .T. ) ;
#7357=CARTESIAN_POINT ( 'NONE',  ( 19.56809120928344825, -8.974600000000002353, 5.000000000000079936 ) ) ;
#7358=ORIENTED_EDGE ( 'NONE', *, *, #5696, .T. ) ;
#7365=EDGE_CURVE ( 'NONE', #14744, #5198, #9707, .T. ) ;
#7369=ADVANCED_FACE ( 'NONE', ( #15220 ), #21039, .F. ) ;
#7375=ORIENTED_EDGE ( 'NONE', *, *, #20158, .F. ) ;
#7383=ORIENTED_EDGE ( 'NONE', *, *, #18009, .F. ) ;
#7389=DIRECTION ( 'NONE',  ( 1.000000000000000000, 7.703719777548943412E-32, 0.000000000000000000 ) ) ;
#7393=PLANE ( 'NONE',  #14942 ) ;
#7398=LINE ( 'NONE', #3654, #19089 ) ;
#7401=ORIENTED_EDGE ( 'NONE', *, *, #22798, .F. ) ;
#7402=CARTESIAN_POINT ( 'NONE',  ( 18.97172504071656363, -8.974600000000002353, 5.000000000000079936 ) ) ;
#7408=ORIENTED_EDGE ( 'NONE', *, *, #3373, .T. ) ;
#7410=VERTEX_POINT ( 'NONE', #8262 ) ;
#7412=ORIENTED_EDGE ( 'NONE', *, *, #15246, .T. ) ;
#7418=CARTESIAN_POINT ( 'NONE',  ( 118.3095189484530181, -7.098169556225942145, 56.71010071662853136 ) ) ;
#7432=ORIENTED_EDGE ( 'NONE', *, *, #8689, .T. ) ;
#7433=DIRECTION ( 'NONE',  ( 0.3420201433256622736, -0.9396926207859106484, -1.232595164407828100E-31 ) ) ;
#7447=VERTEX_POINT ( 'NONE', #21629 ) ;
#7458=ORIENTED_EDGE ( 'NONE', *, *, #1427, .F. ) ;
#7460=VERTEX_POINT ( 'NONE', #14125 ) ;
#7470=AXIS2_PLACEMENT_3D ( 'NONE', #23318, #6926, #14243 ) ;
#7480=CARTESIAN_POINT ( 'NONE',  ( 14.11308378033275446, -11.25000000000000355, 10.00000000000008882 ) ) ;
#7484=ORIENTED_EDGE ( 'NONE', *, *, #19484, .T. ) ;
#7487=ORIENTED_EDGE ( 'NONE', *, *, #5850, .F. ) ;
#7498=CARTESIAN_POINT ( 'NONE',  ( -0.7060087303327398089, -11.25000000000000355, 5.000000000000079936 ) ) ;
#7499=ORIENTED_EDGE ( 'NONE', *, *, #1162, .F. ) ;
#7504=AXIS2_PLACEMENT_3D ( 'NONE', #14662, #21919, #2043 ) ;
#7512=LINE ( 'NONE', #2089, #14170 ) ;
#7514=LINE ( 'NONE', #4138, #3279 ) ;
#7518=DIRECTION ( 'NONE',  ( 0.3420201433256622736, 0.9396926207859106484, 0.000000000000000000 ) ) ;
#7529=EDGE_CURVE ( 'NONE', #17653, #18371, #15807, .T. ) ;
#7530=CARTESIAN_POINT ( 'NONE',  ( -19.99999999999999645, -9.000000000000003553, 5.000000000000079936 ) ) ;
#7536=DIRECTION ( 'NONE',  ( 1.000000000000000000, 7.703719777548943412E-32, 0.000000000000000000 ) ) ;
#7544=ORIENTED_EDGE ( 'NONE', *, *, #19308, .F. ) ;
#7545=LINE ( 'NONE', #23587, #20070 ) ;
#7546=CARTESIAN_POINT ( 'NONE',  ( 47.23681404676619877, -9.000000000000001776, 10.00000000000008882 ) ) ;
#7552=FACE_OUTER_BOUND ( 'NONE', #3120, .T. ) ;
#7563=VECTOR ( 'NONE', #168, 1000.000000000000114 ) ;
#7569=ADVANCED_FACE ( 'NONE', ( #10544 ), #21390, .F. ) ;
#7574=FACE_OUTER_BOUND ( 'NONE', #1581, .T. ) ;
#7578=ORIENTED_EDGE ( 'NONE', *, *, #4930, .F. ) ;
#7582=CARTESIAN_POINT ( 'NONE',  ( 7.001720609283449193, -8.974600000000002353, 5.000000000000079936 ) ) ;
#7583=EDGE_LOOP ( 'NONE', ( #7401, #6309, #23451, #19227 ) ) ;
#7585=VECTOR ( 'NONE', #23495, 1000.000000000000114 ) ;
#7592=LINE ( 'NONE', #14914, #378 ) ;
#7604=ORIENTED_EDGE ( 'NONE', *, *, #11605, .F. ) ;
#7607=ORIENTED_EDGE ( 'NONE', *, *, #22460, .T. ) ;
#7615=CARTESIAN_POINT ( 'NONE',  ( -19.99999999999999645, -15.00000000000001954, 5.000000000000079936 ) ) ;
#7618=PRODUCT_DEFINITION_SHAPE ( 'NONE', 'NONE',  #2996 ) ;
#7622=EDGE_CURVE ( 'NONE', #21366, #6714, #20780, .T. ) ;
#7623=VECTOR ( 'NONE', #1204, 999.9999999999998863 ) ;
#7624=CARTESIAN_POINT ( 'NONE',  ( 118.3095189484530181, -10.00000000000001954, 15.00000000000002842 ) ) ;
#7628=EDGE_CURVE ( 'NONE', #22527, #6569, #6313, .T. ) ;
#7635=ORIENTED_EDGE ( 'NONE', *, *, #6308, .F. ) ;
#7636=DIRECTION ( 'NONE',  ( 0.9396926207859107594, -0.3420201433256623291, 3.697785493223492838E-32 ) ) ;
#7637=AXIS2_PLACEMENT_3D ( 'NONE', #9202, #6919, #20167 ) ;
#7640=ADVANCED_FACE ( 'NONE', ( #4501 ), #8125, .F. ) ;
#7645=AXIS2_PLACEMENT_3D ( 'NONE', #2964, #13789, #8511 ) ;
#7648=CARTESIAN_POINT ( 'NONE',  ( 12.67929489676620314, -9.000000000000005329, 10.00000000000008882 ) ) ;
#7659=CARTESIAN_POINT ( 'NONE',  ( 45.00000000000000000, -9.796556200126378400, 10.00000000000008882 ) ) ;
#7663=CARTESIAN_POINT ( 'NONE',  ( 8.718769219667262149, -11.25000000000000355, 5.000000000000079936 ) ) ;
#7675=LINE ( 'NONE', #21890, #5932 ) ;
#7676=DIRECTION ( 'NONE',  ( 7.087422195345011518E-32, 1.000000000000000000, -0.000000000000000000 ) ) ;
#7678=VECTOR ( 'NONE', #20739, 1000.000000000000000 ) ;
#7680=VERTEX_POINT ( 'NONE', #15320 ) ;
#7687=CARTESIAN_POINT ( 'NONE',  ( 25.25491034071656316, -8.974600000000002353, 5.000000000000079936 ) ) ;
#7696=FACE_OUTER_BOUND ( 'NONE', #18578, .T. ) ;
#7708=ORIENTED_EDGE ( 'NONE', *, *, #8808, .F. ) ;
#7712=VERTEX_POINT ( 'NONE', #6067 ) ;
#7715=ADVANCED_FACE ( 'NONE', ( #21479 ), #15668, .F. ) ;
#7725=DIRECTION ( 'NONE',  ( 0.3420201433256622181, 0.9396926207859107594, -6.162975822039141593E-32 ) ) ;
#7727=CARTESIAN_POINT ( 'NONE',  ( 33.85151041966726382, -11.25000000000000355, 10.00000000000008882 ) ) ;
#7728=ORIENTED_EDGE ( 'NONE', *, *, #441, .T. ) ;
#7739=ORIENTED_EDGE ( 'NONE', *, *, #3220, .F. ) ;
#7742=EDGE_CURVE ( 'NONE', #6426, #6127, #19690, .T. ) ;
#7765=EDGE_CURVE ( 'NONE', #5838, #6808, #3171, .T. ) ;
#7766=EDGE_CURVE ( 'NONE', #3172, #13557, #7019, .T. ) ;
#7777=DIRECTION ( 'NONE',  ( 0.000000000000000000, 0.000000000000000000, -1.000000000000000000 ) ) ;
#7783=DIRECTION ( 'NONE',  ( -1.000000000000000000, -7.703719777548943412E-32, 0.000000000000000000 ) ) ;
#7792=DIRECTION ( 'NONE',  ( 0.000000000000000000, 0.000000000000000000, -1.000000000000000000 ) ) ;
#7794=CARTESIAN_POINT ( 'NONE',  ( -12.44420145928343935, -8.974600000000002353, 10.00000000000008882 ) ) ;
#7801=EDGE_CURVE ( 'NONE', #7712, #1981, #5210, .T. ) ;
#7810=CARTESIAN_POINT ( 'NONE',  ( -19.99999999999999645, -9.000000000000003553, 10.00000000000008882 ) ) ;
#7829=DIRECTION ( 'NONE',  ( 0.000000000000000000, 0.000000000000000000, -1.000000000000000000 ) ) ;
#7837=DIRECTION ( 'NONE',  ( -7.087422195345011518E-32, -1.000000000000000000, 0.000000000000000000 ) ) ;
#7844=DIRECTION ( 'NONE',  ( -5.546678239835226120E-32, -0.3420201433256691015, -0.9396926207859083169 ) ) ;
#7845=VECTOR ( 'NONE', #7837, 1000.000000000000000 ) ;
#7847=DIRECTION ( 'NONE',  ( 0.9396926207859107594, -0.3420201433256623291, 3.697785493223492838E-32 ) ) ;
#7853=CARTESIAN_POINT ( 'NONE',  ( 50.00000000000000000, -10.00000000000001954, 17.50000000000002842 ) ) ;
#7854=VECTOR ( 'NONE', #16526, 1000.000000000000000 ) ;
#7860=DIRECTION ( 'NONE',  ( 0.3420201433256622736, -0.9396926207859106484, -1.232595164407828100E-31 ) ) ;
#7873=ORIENTED_EDGE ( 'NONE', *, *, #119, .T. ) ;
#7886=LINE ( 'NONE', #6080, #1175 ) ;
#7891=ORIENTED_EDGE ( 'NONE', *, *, #1001, .F. ) ;
#7893=ORIENTED_EDGE ( 'NONE', *, *, #13145, .F. ) ;
#7903=ORIENTED_EDGE ( 'NONE', *, *, #22798, .T. ) ;
#7904=CARTESIAN_POINT ( 'NONE',  ( 50.00000000000000000, -2.399706452296379577, 55.00000000000021316 ) ) ;
#7905=ORIENTED_EDGE ( 'NONE', *, *, #20638, .T. ) ;
#7909=FACE_OUTER_BOUND ( 'NONE', #18640, .T. ) ;
#7910=ORIENTED_EDGE ( 'NONE', *, *, #8797, .F. ) ;
#7911=CARTESIAN_POINT ( 'NONE',  ( 118.3095189484530181, -2.399706452296352932, 60.00000000000021316 ) ) ;
#7914=ORIENTED_EDGE ( 'NONE', *, *, #20670, .T. ) ;
#7916=ADVANCED_FACE ( 'NONE', ( #12551 ), #23530, .F. ) ;
#7923=ADVANCED_FACE ( 'NONE', ( #19813 ), #16241, .F. ) ;
#7936=DIRECTION ( 'NONE',  ( 0.3420201433256622181, 0.9396926207859107594, -6.162975822039141593E-32 ) ) ;
#7948=CARTESIAN_POINT ( 'NONE',  ( -2.423057340716551433, -8.974600000000002353, 5.000000000000079936 ) ) ;
#7956=VECTOR ( 'NONE', #5008, 1000.000000000000000 ) ;
#7997=CARTESIAN_POINT ( 'NONE',  ( 1.077186599943259049, -1.328531455546325901, 10.00000000000008882 ) ) ;
#8013=CARTESIAN_POINT ( 'NONE',  ( -11.83859044676619199, -9.000000000000003553, 5.000000000000079936 ) ) ;
#8018=FACE_OUTER_BOUND ( 'NONE', #16472, .T. ) ;
#8022=DIRECTION ( 'NONE',  ( -1.000000000000000000, -7.703719777548943412E-32, 0.000000000000000000 ) ) ;
#8023=DIRECTION ( 'NONE',  ( 0.3420201433256622181, 0.9396926207859107594, -6.162975822039141593E-32 ) ) ;
#8035=EDGE_CURVE ( 'NONE', #4570, #21726, #13016, .T. ) ;
#8043=VECTOR ( 'NONE', #8110, 1000.000000000000000 ) ;
#8044=CARTESIAN_POINT ( 'NONE',  ( 11.86036186966726191, -11.25000000000000355, 5.000000000000079936 ) ) ;
#8046=EDGE_CURVE ( 'NONE', #13738, #12252, #280, .T. ) ;
#8050=DIRECTION ( 'NONE',  ( 7.087422195345011518E-32, 1.000000000000000000, 0.000000000000000000 ) ) ;
#8052=ORIENTED_EDGE ( 'NONE', *, *, #20012, .F. ) ;
#8056=CARTESIAN_POINT ( 'NONE',  ( 29.82104703033275328, -11.25000000000000355, 10.00000000000008882 ) ) ;
#8059=ORIENTED_EDGE ( 'NONE', *, *, #14106, .T. ) ;
#8063=ORIENTED_EDGE ( 'NONE', *, *, #5397, .F. ) ;
#8089=FACE_BOUND ( 'NONE', #9446, .T. ) ;
#8090=ORIENTED_EDGE ( 'NONE', *, *, #1290, .F. ) ;
#8097=FACE_OUTER_BOUND ( 'NONE', #2286, .T. ) ;
#8101=EDGE_CURVE ( 'NONE', #17388, #5511, #5806, .T. ) ;
#8105=ADVANCED_FACE ( 'NONE', ( #8097 ), #526, .F. ) ;
#8110=DIRECTION ( 'NONE',  ( -1.000000000000000000, -7.703719777548943412E-32, 0.000000000000000000 ) ) ;
#8116=LINE ( 'NONE', #15660, #2021 ) ;
#8118=ORIENTED_EDGE ( 'NONE', *, *, #14745, .F. ) ;
#8120=DIRECTION ( 'NONE',  ( 0.3420201433256622181, -0.9396926207859107594, 0.000000000000000000 ) ) ;
#8123=ORIENTED_EDGE ( 'NONE', *, *, #20956, .T. ) ;
#8125=PLANE ( 'NONE',  #11802 ) ;
#8141=DIRECTION ( 'NONE',  ( -7.087422195345011518E-32, -1.000000000000000000, -0.000000000000000000 ) ) ;
#8142=CARTESIAN_POINT ( 'NONE',  ( -19.99999999999999645, -9.000000000000003553, 10.00000000000008882 ) ) ;
#8144=CARTESIAN_POINT ( 'NONE',  ( -19.99999999999999645, -9.000000000000003553, 10.00000000000008882 ) ) ;
#8148=PLANE ( 'NONE',  #9501 ) ;
#8152=CARTESIAN_POINT ( 'NONE',  ( -19.99999999999999645, -11.25000000000000355, 5.000000000000079936 ) ) ;
#8156=DIRECTION ( 'NONE',  ( 0.000000000000000000, 0.000000000000000000, 1.000000000000000000 ) ) ;
#8157=CARTESIAN_POINT ( 'NONE',  ( 7.829898480332751376, -11.25000000000000355, 5.000000000000079936 ) ) ;
#8164=CARTESIAN_POINT ( 'NONE',  ( 40.13469571966727045, -11.25000000000000355, 5.000000000000079936 ) ) ;
#8165=ORIENTED_EDGE ( 'NONE', *, *, #11151, .T. ) ;
#8187=CARTESIAN_POINT ( 'NONE',  ( 7.001720609283449193, -8.974600000000002353, 5.000000000000079936 ) ) ;
#8196=EDGE_CURVE ( 'NONE', #23499, #10094, #4356, .T. ) ;
#8216=CARTESIAN_POINT ( 'NONE',  ( 45.00000000000000000, -2.399706452296379577, 55.00000000000021316 ) ) ;
#8235=LINE ( 'NONE', #13513, #3335 ) ;
#8258=DIRECTION ( 'NONE',  ( 0.9396926207859107594, -0.3420201433256623291, 3.697785493223492838E-32 ) ) ;
#8262=CARTESIAN_POINT ( 'NONE',  ( -9.311853653233800543, -9.000000000000005329, 5.000000000000079936 ) ) ;
#8265=EDGE_LOOP ( 'NONE', ( #17214, #12442, #12273, #7073 ) ) ;
#8266=ADVANCED_FACE ( 'NONE', ( #15975 ), #10611, .F. ) ;
#8269=AXIS2_PLACEMENT_3D ( 'NONE', #11033, #3821, #16889 ) ;
#8286=DIRECTION ( 'NONE',  ( -1.000000000000000000, -7.703719777548943412E-32, 0.000000000000000000 ) ) ;
#8291=DIRECTION ( 'NONE',  ( 0.3420201433256622181, 0.9396926207859107594, -6.162975822039141593E-32 ) ) ;
#8292=EDGE_LOOP ( 'NONE', ( #4511, #22396, #11863, #7893 ) ) ;
#8297=DIRECTION ( 'NONE',  ( 0.000000000000000000, 0.000000000000000000, -1.000000000000000000 ) ) ;
#8300=CARTESIAN_POINT ( 'NONE',  ( 48.67060293033276963, -11.25000000000000355, 5.000000000000079936 ) ) ;
#8306=CARTESIAN_POINT ( 'NONE',  ( -19.99999999999999645, -9.000000000000003553, 5.000000000000079936 ) ) ;
#8315=VERTEX_POINT ( 'NONE', #21212 ) ;
#8332=VECTOR ( 'NONE', #12577, 1000.000000000000000 ) ;
#8343=ORIENTED_EDGE ( 'NONE', *, *, #11733, .T. ) ;
#8372=PLANE ( 'NONE',  #14787 ) ;
#8380=DIRECTION ( 'NONE',  ( 0.3420201433256622736, -0.9396926207859106484, -1.232595164407828100E-31 ) ) ;
#8382=CARTESIAN_POINT ( 'NONE',  ( 33.85151041966726382, -11.25000000000000355, 10.00000000000008882 ) ) ;
#8383=ORIENTED_EDGE ( 'NONE', *, *, #22970, .T. ) ;
#8425=CARTESIAN_POINT ( 'NONE',  ( -3.847601380332740018, -11.25000000000000355, 10.00000000000008882 ) ) ;
#8438=AXIS2_PLACEMENT_3D ( 'NONE', #507, #20496, #7829 ) ;
#8446=VERTEX_POINT ( 'NONE', #2046 ) ;
#8456=CARTESIAN_POINT ( 'NONE',  ( 31.53809564071656624, -8.974600000000002353, 5.000000000000079936 ) ) ;
#8479=CARTESIAN_POINT ( 'NONE',  ( 45.00000000000000000, 2.399706452296353820, 60.00000000000021316 ) ) ;
#8480=CARTESIAN_POINT ( 'NONE',  ( -4.736472119667250347, -11.25000000000000355, 5.000000000000079936 ) ) ;
#8482=CARTESIAN_POINT ( 'NONE',  ( 118.3095189484530181, -10.00000000000001954, 17.50000000000003553 ) ) ;
#8483=AXIS2_PLACEMENT_3D ( 'NONE', #19618, #14384, #15823 ) ;
#8492=DIRECTION ( 'NONE',  ( 1.000000000000000000, 7.703719777548943412E-32, 0.000000000000000000 ) ) ;
#8504=ORIENTED_EDGE ( 'NONE', *, *, #18112, .T. ) ;
#8507=FACE_OUTER_BOUND ( 'NONE', #23110, .T. ) ;
#8511=DIRECTION ( 'NONE',  ( 0.000000000000000000, 0.000000000000000000, -1.000000000000000000 ) ) ;
#8516=DIRECTION ( 'NONE',  ( 0.9396926207859107594, -0.3420201433256623291, 3.697785493223492838E-32 ) ) ;
#8519=DIRECTION ( 'NONE',  ( 1.000000000000000000, 7.703719777548943412E-32, 0.000000000000000000 ) ) ;
#8522=LINE ( 'NONE', #6710, #15920 ) ;
#8555=VECTOR ( 'NONE', #13852, 1000.000000000000000 ) ;
#8559=ORIENTED_EDGE ( 'NONE', *, *, #7202, .F. ) ;
#8560=EDGE_CURVE ( 'NONE', #19450, #15217, #3174, .T. ) ;
#8563=PLANE ( 'NONE',  #19771 ) ;
#8577=CARTESIAN_POINT ( 'NONE',  ( 8.718769219667262149, -11.25000000000000355, 10.00000000000008882 ) ) ;
#8582=ORIENTED_EDGE ( 'NONE', *, *, #21922, .T. ) ;
#8586=VERTEX_POINT ( 'NONE', #21602 ) ;
#8587=DIRECTION ( 'NONE',  ( 0.000000000000000000, 0.000000000000000000, -1.000000000000000000 ) ) ;
#8601=ORIENTED_EDGE ( 'NONE', *, *, #10989, .T. ) ;
#8603=CARTESIAN_POINT ( 'NONE',  ( -0.7060087303327398089, -11.25000000000000355, 5.000000000000079936 ) ) ;
#8606=ORIENTED_EDGE ( 'NONE', *, *, #23226, .F. ) ;
#8610=EDGE_LOOP ( 'NONE', ( #18545, #13511, #18789, #16045 ) ) ;
#8623=EDGE_CURVE ( 'NONE', #22275, #5838, #11755, .T. ) ;
#8630=EDGE_LOOP ( 'NONE', ( #20970, #22871, #1754, #20796 ) ) ;
#8640=VERTEX_POINT ( 'NONE', #6781 ) ;
#8641=FACE_OUTER_BOUND ( 'NONE', #22582, .T. ) ;
#8646=DIRECTION ( 'NONE',  ( 1.000000000000000000, 7.703719777548943412E-32, 0.000000000000000000 ) ) ;
#8648=VECTOR ( 'NONE', #4201, 1000.000000000000000 ) ;
#8653=CARTESIAN_POINT ( 'NONE',  ( 5.577176569667260608, -11.25000000000000355, 5.000000000000079936 ) ) ;
#8656=CARTESIAN_POINT ( 'NONE',  ( 50.00000000000000000, 14.69846310392956745, 35.82846581308617573 ) ) ;
#8666=CARTESIAN_POINT ( 'NONE',  ( 45.00000000000000000, -2.399706452296378245, 55.00000000000021316 ) ) ;
#8680=DIRECTION ( 'NONE',  ( 7.087422195345011518E-32, 1.000000000000000000, -0.000000000000000000 ) ) ;
#8689=EDGE_CURVE ( 'NONE', #12712, #10456, #22065, .T. ) ;
#8691=EDGE_CURVE ( 'NONE', #11492, #4376, #17972, .T. ) ;
#8692=ORIENTED_EDGE ( 'NONE', *, *, #21456, .F. ) ;
#8696=DIRECTION ( 'NONE',  ( -7.703719777548925896E-32, -0.9396926207859083169, -0.3420201433256691015 ) ) ;
#8698=DIRECTION ( 'NONE',  ( -7.087422195345011518E-32, -1.000000000000000000, -0.000000000000000000 ) ) ;
#8707=CARTESIAN_POINT ( 'NONE',  ( -3.847601380332740018, -11.25000000000000355, 5.000000000000079936 ) ) ;
#8709=AXIS2_PLACEMENT_3D ( 'NONE', #13694, #23009, #10463 ) ;
#8724=ORIENTED_EDGE ( 'NONE', *, *, #9943, .T. ) ;
#8725=CARTESIAN_POINT ( 'NONE',  ( 45.00000000000000000, 7.098169556225943033, 56.71010071662853136 ) ) ;
#8729=LINE ( 'NONE', #15699, #8763 ) ;
#8738=VERTEX_POINT ( 'NONE', #20282 ) ;
#8746=DIRECTION ( 'NONE',  ( 1.000000000000000000, 7.703719777548943412E-32, 0.000000000000000000 ) ) ;
#8747=LINE ( 'NONE', #12357, #19175 ) ;
#8754=VECTOR ( 'NONE', #8868, 1000.000000000000000 ) ;
#8757=DIRECTION ( 'NONE',  ( 1.000000000000000000, 7.703719777548943412E-32, 0.000000000000000000 ) ) ;
#8758=ORIENTED_EDGE ( 'NONE', *, *, #4797, .F. ) ;
#8760=ORIENTED_EDGE ( 'NONE', *, *, #19578, .F. ) ;
#8763=VECTOR ( 'NONE', #12454, 1000.000000000000114 ) ;
#8780=CARTESIAN_POINT ( 'NONE',  ( 15.00195451966726523, -11.25000000000000355, 5.000000000000079936 ) ) ;
#8792=VECTOR ( 'NONE', #14011, 1000.000000000000000 ) ;
#8797=EDGE_CURVE ( 'NONE', #1835, #6127, #56, .T. ) ;
#8798=EDGE_CURVE ( 'NONE', #10010, #2729, #14698, .T. ) ;
#8808=EDGE_CURVE ( 'NONE', #9681, #5198, #5683, .T. ) ;
#8809=CARTESIAN_POINT ( 'NONE',  ( 31.52885079676620705, -9.000000000000005329, 5.000000000000079936 ) ) ;
#8828=VERTEX_POINT ( 'NONE', #18494 ) ;
#8839=ORIENTED_EDGE ( 'NONE', *, *, #14508, .T. ) ;
#8856=ORIENTED_EDGE ( 'NONE', *, *, #10982, .T. ) ;
#8857=CARTESIAN_POINT ( 'NONE',  ( -10.13078668033273999, -11.25000000000000355, 5.000000000000079936 ) ) ;
#8866=DIRECTION ( 'NONE',  ( -1.848892746611741766E-32, -0.3420201433256689905, 0.9396926207859082059 ) ) ;
#8868=DIRECTION ( 'NONE',  ( -1.000000000000000000, -7.703719777548943412E-32, 0.000000000000000000 ) ) ;
#8869=ORIENTED_EDGE ( 'NONE', *, *, #20605, .F. ) ;
#8870=VECTOR ( 'NONE', #21770, 1000.000000000000000 ) ;
#8890=CARTESIAN_POINT ( 'NONE',  ( -15.56739012628458774, -7.386661945853154165, 10.00000000000008882 ) ) ;
#8895=CARTESIAN_POINT ( 'NONE',  ( 32.14370665323380649, -9.000000000000001776, 5.000000000000079936 ) ) ;
#8916=DIRECTION ( 'NONE',  ( 0.9396926207859107594, -0.3420201433256623291, 3.697785493223492838E-32 ) ) ;
#8924=FACE_OUTER_BOUND ( 'NONE', #7058, .T. ) ;
#8930=ADVANCED_FACE ( 'NONE', ( #11911 ), #22886, .F. ) ;
#8945=EDGE_CURVE ( 'NONE', #6808, #17107, #2763, .T. ) ;
#8946=CARTESIAN_POINT ( 'NONE',  ( -9.302608809283439584, -8.974600000000002353, 5.000000000000079936 ) ) ;
#8953=ORIENTED_EDGE ( 'NONE', *, *, #13250, .T. ) ;
#8954=LINE ( 'NONE', #12895, #349 ) ;
#8960=EDGE_CURVE ( 'NONE', #15223, #6641, #4686, .T. ) ;
#8961=CARTESIAN_POINT ( 'NONE',  ( 37.14043617343693171, 11.79741794011847311, 10.00000000000008882 ) ) ;
#8964=EDGE_CURVE ( 'NONE', #13557, #2919, #21427, .T. ) ;
#8966=SURFACE_STYLE_USAGE ( .BOTH. , #5461 ) ;
#8976=EDGE_CURVE ( 'NONE', #8586, #16559, #12259, .T. ) ;
#8988=DIRECTION ( 'NONE',  ( 0.3420201433256622736, 0.9396926207859106484, 0.000000000000000000 ) ) ;
#9006=LINE ( 'NONE', #19978, #7854 ) ;
#9008=DIRECTION ( 'NONE',  ( 1.000000000000000000, 7.703719777548943412E-32, 0.000000000000000000 ) ) ;
#9020=VECTOR ( 'NONE', #19946, 1000.000000000000000 ) ;
#9021=CARTESIAN_POINT ( 'NONE',  ( -19.99999999999999645, -9.000000000000003553, 10.00000000000008882 ) ) ;
#9028=LINE ( 'NONE', #21556, #3067 ) ;
#9029=VERTEX_POINT ( 'NONE', #10698 ) ;
#9036=AXIS2_PLACEMENT_3D ( 'NONE', #22523, #6492, #11903 ) ;
#9040=EDGE_CURVE ( 'NONE', #13240, #22158, #23476, .T. ) ;
#9051=FACE_OUTER_BOUND ( 'NONE', #11548, .T. ) ;
#9063=DIRECTION ( 'NONE',  ( 0.000000000000000000, 0.000000000000000000, -1.000000000000000000 ) ) ;
#9065=ORIENTED_EDGE ( 'NONE', *, *, #5667, .F. ) ;
#9066=CARTESIAN_POINT ( 'NONE',  ( -17.30284271966725029, -11.25000000000000355, 10.00000000000008882 ) ) ;
#9078=LINE ( 'NONE', #10879, #17946 ) ;
#9080=VECTOR ( 'NONE', #1674, 1000.000000000000000 ) ;
#9084=CARTESIAN_POINT ( 'NONE',  ( 44.10446624071656174, -8.974600000000002353, 5.000000000000079936 ) ) ;
#9085=DIRECTION ( 'NONE',  ( -1.000000000000000000, -7.703719777548943412E-32, 0.000000000000000000 ) ) ;
#9095=EDGE_CURVE ( 'NONE', #21366, #17500, #7085, .T. ) ;
#9097=CARTESIAN_POINT ( 'NONE',  ( -10.01919788420863711, -5.367285115750873636, 10.00000000000008882 ) ) ;
#9104=VECTOR ( 'NONE', #19581, 1000.000000000000000 ) ;
#9105=DIRECTION ( 'NONE',  ( 0.000000000000000000, 0.000000000000000000, 1.000000000000000000 ) ) ;
#9108=DIRECTION ( 'NONE',  ( -7.087422195345011518E-32, -1.000000000000000000, -0.000000000000000000 ) ) ;
#9117=DIRECTION ( 'NONE',  ( 0.3420201433256622181, 0.9396926207859107594, -6.162975822039141593E-32 ) ) ;
#9119=ORIENTED_EDGE ( 'NONE', *, *, #16704, .F. ) ;
#9120=LINE ( 'NONE', #14514, #10564 ) ;
#9132=VECTOR ( 'NONE', #1218, 1000.000000000000000 ) ;
#9134=EDGE_CURVE ( 'NONE', #6815, #4263, #1673, .T. ) ;
#9135=CARTESIAN_POINT ( 'NONE',  ( 22.10407284676620066, -9.000000000000001776, 5.000000000000079936 ) ) ;
#9138=EDGE_CURVE ( 'NONE', #13563, #6932, #9252, .T. ) ;
#9158=ORIENTED_EDGE ( 'NONE', *, *, #13888, .T. ) ;
#9161=VECTOR ( 'NONE', #5280, 1000.000000000000000 ) ;
#9169=DIRECTION ( 'NONE',  ( 1.000000000000000000, 7.703719777548943412E-32, 0.000000000000000000 ) ) ;
#9177=VECTOR ( 'NONE', #12820, 1000.000000000000000 ) ;
#9193=VECTOR ( 'NONE', #12926, 1000.000000000000114 ) ;
#9202=CARTESIAN_POINT ( 'NONE',  ( 45.00000000000000000, 2.399706452296377801, 55.00000000000021316 ) ) ;
#9206=ORIENTED_EDGE ( 'NONE', *, *, #11731, .T. ) ;
#9214=ADVANCED_FACE ( 'NONE', ( #13194 ), #14879, .T. ) ;
#9219=VECTOR ( 'NONE', #18051, 1000.000000000000114 ) ;
#9230=LINE ( 'NONE', #9451, #7069 ) ;
#9231=LINE ( 'NONE', #16517, #12835 ) ;
#9233=LINE ( 'NONE', #16401, #10369 ) ;
#9239=ORIENTED_EDGE ( 'NONE', *, *, #20791, .T. ) ;
#9242=LINE ( 'NONE', #22125, #15550 ) ;
#9247=ADVANCED_FACE ( 'NONE', ( #15354 ), #13082, .F. ) ;
#9251=VECTOR ( 'NONE', #561, 1000.000000000000000 ) ;
#9252=LINE ( 'NONE', #20222, #750 ) ;
#9260=PLANE ( 'NONE',  #10361 ) ;
#9262=EDGE_CURVE ( 'NONE', #4473, #2044, #11757, .T. ) ;
#9263=CARTESIAN_POINT ( 'NONE',  ( 44.70083240928345703, -8.974600000000002353, 5.000000000000079936 ) ) ;
#9286=CARTESIAN_POINT ( 'NONE',  ( -19.99999999999999645, -9.000000000000003553, 5.000000000000079936 ) ) ;
#9299=DIRECTION ( 'NONE',  ( -0.3420201433256622181, 0.9396926207859106484, 1.232595164407828100E-31 ) ) ;
#9302=LINE ( 'NONE', #16132, #14912 ) ;
#9312=DIRECTION ( 'NONE',  ( 1.000000000000000000, 7.703719777548943412E-32, 0.000000000000000000 ) ) ;
#9323=DIRECTION ( 'NONE',  ( -1.000000000000000000, -7.703719777548943412E-32, 0.000000000000000000 ) ) ;
#9333=ORIENTED_EDGE ( 'NONE', *, *, #5557, .T. ) ;
#9335=DIRECTION ( 'NONE',  ( 1.000000000000000000, 7.703719777548943412E-32, 0.000000000000000000 ) ) ;
#9341=VECTOR ( 'NONE', #18971, 1000.000000000000000 ) ;
#9343=ORIENTED_EDGE ( 'NONE', *, *, #10164, .F. ) ;
#9348=PLANE ( 'NONE',  #5159 ) ;
#9351=DIRECTION ( 'NONE',  ( 0.3420201433256622181, -0.9396926207859107594, 0.000000000000000000 ) ) ;
#9360=EDGE_CURVE ( 'NONE', #19331, #23136, #18678, .T. ) ;
#9364=DIRECTION ( 'NONE',  ( 0.000000000000000000, 0.000000000000000000, 1.000000000000000000 ) ) ;
#9378=ORIENTED_EDGE ( 'NONE', *, *, #10409, .T. ) ;
#9382=CARTESIAN_POINT ( 'NONE',  ( 17.72176332617111072, 4.729599034760502363, 10.00000000000008882 ) ) ;
#9385=VERTEX_POINT ( 'NONE', #19496 ) ;
#9394=EDGE_CURVE ( 'NONE', #15051, #10887, #21157, .T. ) ;
#9402=VERTEX_POINT ( 'NONE', #19147 ) ;
#9407=CIRCLE ( 'NONE', #7504, 5.000000000000011546 ) ;
#9410=PLANE ( 'NONE',  #9799 ) ;
#9421=ADVANCED_FACE ( 'NONE', ( #3207 ), #1052, .T. ) ;
#9422=DIRECTION ( 'NONE',  ( 0.3420201433256622736, -0.9396926207859106484, -1.232595164407828100E-31 ) ) ;
#9443=LINE ( 'NONE', #7530, #22565 ) ;
#9446=EDGE_LOOP ( 'NONE', ( #6837, #9158 ) ) ;
#9450=DIRECTION ( 'NONE',  ( 0.3420201433256622736, -0.9396926207859106484, -1.232595164407828100E-31 ) ) ;
#9451=CARTESIAN_POINT ( 'NONE',  ( 34.67044344676619971, -9.000000000000003553, 5.000000000000079936 ) ) ;
#9459=( NAMED_UNIT ( * ) SI_UNIT ( $, .STERADIAN. ) SOLID_ANGLE_UNIT ( ) );
#9460=ORIENTED_EDGE ( 'NONE', *, *, #4072, .T. ) ;
#9463=PLANE ( 'NONE',  #17167 ) ;
#9476=ORIENTED_EDGE ( 'NONE', *, *, #3933, .T. ) ;
#9478=DIRECTION ( 'NONE',  ( 1.000000000000000000, 7.703719777548943412E-32, 0.000000000000000000 ) ) ;
#9496=EDGE_CURVE ( 'NONE', #22158, #22026, #15466, .T. ) ;
#9497=EDGE_LOOP ( 'NONE', ( #557, #23162, #10513, #20689 ) ) ;
#9498=DIRECTION ( 'NONE',  ( -0.9396926207859107594, -0.3420201433256623291, 1.540743955509804830E-32 ) ) ;
#9501=AXIS2_PLACEMENT_3D ( 'NONE', #15459, #22366, #17002 ) ;
#9512=DIRECTION ( 'NONE',  ( -0.000000000000000000, 0.000000000000000000, -1.000000000000000000 ) ) ;
#9526=ORIENTED_EDGE ( 'NONE', *, *, #5523, .T. ) ;
#9529=EDGE_CURVE ( 'NONE', #5147, #8640, #22138, .T. ) ;
#9530=DIRECTION ( 'NONE',  ( 0.9396926207859107594, -0.3420201433256623291, 3.697785493223492838E-32 ) ) ;
#9533=VECTOR ( 'NONE', #13088, 1000.000000000000000 ) ;
#9534=CARTESIAN_POINT ( 'NONE',  ( 48.67060293033276963, -11.25000000000000355, 5.000000000000079936 ) ) ;
#9540=CARTESIAN_POINT ( 'NONE',  ( 44.71007725323381976, -9.000000000000003553, 10.29587622221672127 ) ) ;
#9541=VECTOR ( 'NONE', #13044, 1000.000000000000114 ) ;
#9545=VECTOR ( 'NONE', #16625, 1000.000000000000000 ) ;
#9546=CARTESIAN_POINT ( 'NONE',  ( 45.00000000000000000, 2.399706452296379577, 55.00000000000021316 ) ) ;
#9558=ADVANCED_FACE ( 'NONE', ( #6941 ), #12585, .F. ) ;
#9562=CARTESIAN_POINT ( 'NONE',  ( 26.67945438033275707, -11.25000000000000355, 5.000000000000079936 ) ) ;
#9563=EDGE_CURVE ( 'NONE', #10094, #2131, #1759, .T. ) ;
#9564=VECTOR ( 'NONE', #19879, 1000.000000000000000 ) ;
#9570=AXIS2_PLACEMENT_3D ( 'NONE', #10053, #17228, #17343 ) ;
#9581=CARTESIAN_POINT ( 'NONE',  ( 15.82088754676620823, -9.000000000000005329, 10.00000000000008882 ) ) ;
#9586=LINE ( 'NONE', #16878, #592 ) ;
#9594=DIRECTION ( 'NONE',  ( 0.000000000000000000, 0.000000000000000000, 1.000000000000000000 ) ) ;
#9597=ADVANCED_FACE ( 'NONE', ( #5125 ), #10789, .F. ) ;
#9609=ORIENTED_EDGE ( 'NONE', *, *, #10101, .F. ) ;
#9611=LINE ( 'NONE', #19032, #11458 ) ;
#9621=CARTESIAN_POINT ( 'NONE',  ( 6.396109596766199168, -9.000000000000005329, 5.000000000000079936 ) ) ;
#9622=ORIENTED_EDGE ( 'NONE', *, *, #3511, .F. ) ;
#9628=ORIENTED_EDGE ( 'NONE', *, *, #2934, .T. ) ;
#9646=DIRECTION ( 'NONE',  ( -7.087422195345011518E-32, -1.000000000000000000, -0.000000000000000000 ) ) ;
#9648=DIRECTION ( 'NONE',  ( 0.000000000000000000, 0.000000000000000000, 1.000000000000000000 ) ) ;
#9653=DIRECTION ( 'NONE',  ( 0.3420201433256622181, -0.9396926207859107594, 0.000000000000000000 ) ) ;
#9656=DIRECTION ( 'NONE',  ( 0.000000000000000000, 0.000000000000000000, 1.000000000000000000 ) ) ;
#9661=EDGE_CURVE ( 'NONE', #8828, #12158, #14492, .T. ) ;
#9665=LINE ( 'NONE', #13608, #18093 ) ;
#9666=DIRECTION ( 'NONE',  ( -1.000000000000000000, -7.703719777548943412E-32, 0.000000000000000000 ) ) ;
#9670=EDGE_CURVE ( 'NONE', #6426, #11370, #21756, .T. ) ;
#9681=VERTEX_POINT ( 'NONE', #5480 ) ;
#9688=ORIENTED_EDGE ( 'NONE', *, *, #20229, .T. ) ;
#9690=LINE ( 'NONE', #672, #338 ) ;
#9698=CARTESIAN_POINT ( 'NONE',  ( 50.00000000000000000, 15.00000000000003375, 55.00000000000021316 ) ) ;
#9701=CARTESIAN_POINT ( 'NONE',  ( 36.10423233033275636, -11.25000000000000355, 10.00000000000008882 ) ) ;
#9704=LINE ( 'NONE', #8144, #22746 ) ;
#9707=LINE ( 'NONE', #6218, #4879 ) ;
#9708=ORIENTED_EDGE ( 'NONE', *, *, #6733, .F. ) ;
#9713=FACE_OUTER_BOUND ( 'NONE', #6213, .T. ) ;
#9718=DIRECTION ( 'NONE',  ( 0.000000000000000000, 0.000000000000000000, -1.000000000000000000 ) ) ;
#9724=DIRECTION ( 'NONE',  ( 0.3420201433256622736, 0.9396926207859106484, 0.000000000000000000 ) ) ;
#9755=ORIENTED_EDGE ( 'NONE', *, *, #22909, .F. ) ;
#9762=ORIENTED_EDGE ( 'NONE', *, *, #10292, .T. ) ;
#9775=CARTESIAN_POINT ( 'NONE',  ( 27.56832511966726784, -11.25000000000000355, 5.000000000000079936 ) ) ;
#9783=CARTESIAN_POINT ( 'NONE',  ( -14.98942794071655271, -8.974600000000002353, 5.000000000000079936 ) ) ;
#9790=ORIENTED_EDGE ( 'NONE', *, *, #18323, .F. ) ;
#9799=AXIS2_PLACEMENT_3D ( 'NONE', #11336, #9530, #21946 ) ;
#9815=DIRECTION ( 'NONE',  ( -1.000000000000000000, -7.703719777548943412E-32, 0.000000000000000000 ) ) ;
#9816=EDGE_CURVE ( 'NONE', #7712, #17107, #9443, .T. ) ;
#9818=ORIENTED_EDGE ( 'NONE', *, *, #22022, .T. ) ;
#9821=LINE ( 'NONE', #4881, #6065 ) ;
#9830=EDGE_CURVE ( 'NONE', #9402, #21235, #16979, .T. ) ;
#9845=DIRECTION ( 'NONE',  ( 0.3420201433256622181, -0.9396926207859107594, 0.000000000000000000 ) ) ;
#9863=VECTOR ( 'NONE', #11520, 1000.000000000000114 ) ;
#9869=CARTESIAN_POINT ( 'NONE',  ( 40.95362874676621345, -9.000000000000005329, 5.000000000000079936 ) ) ;
#9904=CARTESIAN_POINT ( 'NONE',  ( -13.27237933033274153, -11.25000000000000355, 5.000000000000079936 ) ) ;
#9908=DIRECTION ( 'NONE',  ( 7.010384997569516610E-32, 1.000000000000000000, -3.469446951953615175E-16 ) ) ;
#9910=CARTESIAN_POINT ( 'NONE',  ( -18.72738675928344065, -8.974600000000002353, 10.00000000000008882 ) ) ;
#9911=CARTESIAN_POINT ( 'NONE',  ( -19.99999999999999645, -9.000000000000003553, 5.000000000000079936 ) ) ;
#9913=DIRECTION ( 'NONE',  ( 0.000000000000000000, 0.000000000000000000, 1.000000000000000000 ) ) ;
#9918=AXIS2_PLACEMENT_3D ( 'NONE', #12727, #10917, #21418 ) ;
#9922=ORIENTED_EDGE ( 'NONE', *, *, #19154, .F. ) ;
#9931=CIRCLE ( 'NONE', #19473, 5.000000000000011546 ) ;
#9943=EDGE_CURVE ( 'NONE', #8315, #23413, #14434, .T. ) ;
#9950=DIRECTION ( 'NONE',  ( 0.000000000000000000, 0.000000000000000000, -1.000000000000000000 ) ) ;
#9958=DIRECTION ( 'NONE',  ( 0.000000000000000000, 0.000000000000000000, 1.000000000000000000 ) ) ;
#9962=VERTEX_POINT ( 'NONE', #18473 ) ;
#9965=ADVANCED_FACE ( 'NONE', ( #4099 ), #16930, .F. ) ;
#9981=EDGE_LOOP ( 'NONE', ( #10338, #21540, #20634, #2321 ) ) ;
#9985=LINE ( 'NONE', #6133, #10949 ) ;
#9986=EDGE_LOOP ( 'NONE', ( #20862, #2756, #7873, #3696 ) ) ;
#9987=VECTOR ( 'NONE', #22226, 1000.000000000000000 ) ;
#9990=CARTESIAN_POINT ( 'NONE',  ( 45.00000000000000000, 15.00000000000003375, 34.11836509645780069 ) ) ;
#10007=ADVANCED_FACE ( 'NONE', ( #18715 ), #2052, .F. ) ;
#10010=VERTEX_POINT ( 'NONE', #390 ) ;
#10028=DIRECTION ( 'NONE',  ( 1.000000000000000000, 7.703719777548943412E-32, 0.000000000000000000 ) ) ;
#10030=LINE ( 'NONE', #19213, #15711 ) ;
#10037=ADVANCED_FACE ( 'NONE', ( #4225 ), #11561, .F. ) ;
#10052=ORIENTED_EDGE ( 'NONE', *, *, #22460, .F. ) ;
#10053=CARTESIAN_POINT ( 'NONE',  ( 118.3095189484530181, -14.69846310392956745, 35.82846581308617573 ) ) ;
#10055=LINE ( 'NONE', #19238, #9251 ) ;
#10058=CARTESIAN_POINT ( 'NONE',  ( 50.00000000000002132, -10.03966385473554013, 5.000000000000079936 ) ) ;
#10064=CARTESIAN_POINT ( 'NONE',  ( 6.405354440716562792, -8.974600000000002353, 10.00000000000008882 ) ) ;
#10065=CARTESIAN_POINT ( 'NONE',  ( 36.10423233033275636, -11.25000000000000355, 5.000000000000079936 ) ) ;
#10066=CARTESIAN_POINT ( 'NONE',  ( -18.12177574676618974, -9.000000000000003553, 10.00000000000008882 ) ) ;
#10073=VERTEX_POINT ( 'NONE', #1942 ) ;
#10075=DIRECTION ( 'NONE',  ( 0.9396926207859107594, -0.3420201433256623291, 3.697785493223492838E-32 ) ) ;
#10078=CARTESIAN_POINT ( 'NONE',  ( 45.00000000000000000, 10.00000000000001599, 15.00000000000003020 ) ) ;
#10085=LINE ( 'NONE', #22631, #20427 ) ;
#10094=VERTEX_POINT ( 'NONE', #14794 ) ;
#10096=ORIENTED_EDGE ( 'NONE', *, *, #7628, .T. ) ;
#10097=DIRECTION ( 'NONE',  ( -1.000000000000000000, -7.703719777548943412E-32, 0.000000000000000000 ) ) ;
#10098=ORIENTED_EDGE ( 'NONE', *, *, #17341, .T. ) ;
#10101=EDGE_CURVE ( 'NONE', #25, #4980, #7592, .T. ) ;
#10105=VECTOR ( 'NONE', #19973, 1000.000000000000000 ) ;
#10107=CARTESIAN_POINT ( 'NONE',  ( -19.99999999999999645, -9.000000000000003553, 5.000000000000079936 ) ) ;
#10110=LINE ( 'NONE', #8300, #6513 ) ;
#10118=FACE_BOUND ( 'NONE', #13462, .T. ) ;
#10123=EDGE_CURVE ( 'NONE', #14446, #12965, #4454, .T. ) ;
#10128=EDGE_CURVE ( 'NONE', #22239, #4233, #1909, .T. ) ;
#10142=LINE ( 'NONE', #20758, #15843 ) ;
#10159=ORIENTED_EDGE ( 'NONE', *, *, #11605, .T. ) ;
#10162=ORIENTED_EDGE ( 'NONE', *, *, #19308, .T. ) ;
#10164=EDGE_CURVE ( 'NONE', #25, #10781, #1085, .T. ) ;
#10165=EDGE_CURVE ( 'NONE', #6714, #15383, #10110, .T. ) ;
#10172=ORIENTED_EDGE ( 'NONE', *, *, #14552, .T. ) ;
#10173=CARTESIAN_POINT ( 'NONE',  ( 27.56832511966726784, -11.25000000000000355, 10.00000000000008882 ) ) ;
#10181=DIRECTION ( 'NONE',  ( 0.9396926207859107594, -0.3420201433256623291, 3.697785493223492838E-32 ) ) ;
#10186=CIRCLE ( 'NONE', #9036, 2.500000000000007550 ) ;
#10192=LINE ( 'NONE', #8152, #14491 ) ;
#10196=CARTESIAN_POINT ( 'NONE',  ( -17.30284271966725029, -11.25000000000000355, 5.000000000000079936 ) ) ;
#10213=ORIENTED_EDGE ( 'NONE', *, *, #585, .F. ) ;
#10214=DIRECTION ( 'NONE',  ( 0.000000000000000000, 0.000000000000000000, 1.000000000000000000 ) ) ;
#10218=CARTESIAN_POINT ( 'NONE',  ( -8.696997796766190447, -9.000000000000005329, 5.000000000000079936 ) ) ;
#10249=VERTEX_POINT ( 'NONE', #9869 ) ;
#10254=CARTESIAN_POINT ( 'NONE',  ( -3.847601380332740018, -11.25000000000000355, 5.000000000000079936 ) ) ;
#10261=ADVANCED_FACE ( 'NONE', ( #17164 ), #22653, .F. ) ;
#10267=CARTESIAN_POINT ( 'NONE',  ( 25.86052135323381407, -9.000000000000003553, 5.000000000000079936 ) ) ;
#10270=CARTESIAN_POINT ( 'NONE',  ( 0.1129242967662022479, -9.000000000000003553, 5.000000000000079936 ) ) ;
#10272=ORIENTED_EDGE ( 'NONE', *, *, #17715, .F. ) ;
#10275=EDGE_CURVE ( 'NONE', #21235, #14801, #6380, .T. ) ;
#10277=EDGE_CURVE ( 'NONE', #1550, #15217, #12504, .T. ) ;
#10288=LINE ( 'NONE', #8961, #3187 ) ;
#10292=EDGE_CURVE ( 'NONE', #18952, #14717, #14289, .T. ) ;
#10296=DIRECTION ( 'NONE',  ( -7.087422195345011518E-32, -1.000000000000000000, -0.000000000000000000 ) ) ;
#10299=DIRECTION ( 'NONE',  ( -1.000000000000000000, -7.703719777548943412E-32, 0.000000000000000000 ) ) ;
#10305=EDGE_CURVE ( 'NONE', #18509, #23413, #19404, .T. ) ;
#10306=EDGE_LOOP ( 'NONE', ( #7111, #11899, #6928, #6768 ) ) ;
#10310=ORIENTED_EDGE ( 'NONE', *, *, #8035, .F. ) ;
#10312=VERTEX_POINT ( 'NONE', #17750 ) ;
#10322=CARTESIAN_POINT ( 'NONE',  ( 50.00000000000000000, -14.69846310392956745, 35.82846581308617573 ) ) ;
#10323=VECTOR ( 'NONE', #19503, 1000.000000000000114 ) ;
#10333=CARTESIAN_POINT ( 'NONE',  ( 21.28513981966725765, -11.25000000000000355, 10.00000000000008882 ) ) ;
#10338=ORIENTED_EDGE ( 'NONE', *, *, #18852, .T. ) ;
#10344=EDGE_LOOP ( 'NONE', ( #19515, #16183, #10052, #15489 ) ) ;
#10345=ORIENTED_EDGE ( 'NONE', *, *, #14311, .F. ) ;
#10347=AXIS2_PLACEMENT_3D ( 'NONE', #23448, #7304, #8866 ) ;
#10348=CARTESIAN_POINT ( 'NONE',  ( -3.028668353233801458, -9.000000000000005329, 10.00000000000008882 ) ) ;
#10361=AXIS2_PLACEMENT_3D ( 'NONE', #20107, #12743, #16429 ) ;
#10368=ORIENTED_EDGE ( 'NONE', *, *, #2229, .F. ) ;
#10369=VECTOR ( 'NONE', #20084, 1000.000000000000000 ) ;
#10370=CARTESIAN_POINT ( 'NONE',  ( 118.3095189484530181, -15.00000000000003375, 34.11836509645780779 ) ) ;
#10371=VECTOR ( 'NONE', #20941, 1000.000000000000000 ) ;
#10386=DIRECTION ( 'NONE',  ( -7.087422195345011518E-32, -1.000000000000000000, -0.000000000000000000 ) ) ;
#10387=LINE ( 'NONE', #22681, #8043 ) ;
#10392=CARTESIAN_POINT ( 'NONE',  ( 19.57733605323380743, -9.000000000000003553, 5.000000000000079936 ) ) ;
#10394=EDGE_LOOP ( 'NONE', ( #7226, #5011, #5595, #1481 ) ) ;
#10395=DIRECTION ( 'NONE',  ( 0.3420201433256622736, 0.9396926207859106484, 0.000000000000000000 ) ) ;
#10409=EDGE_CURVE ( 'NONE', #8640, #20363, #1433, .T. ) ;
#10410=CARTESIAN_POINT ( 'NONE',  ( -5.555405146766190683, -9.000000000000005329, 10.00000000000008882 ) ) ;
#10419=DIRECTION ( 'NONE',  ( 0.3420201433256622181, 0.9396926207859107594, -6.162975822039141593E-32 ) ) ;
#10425=ORIENTED_EDGE ( 'NONE', *, *, #8798, .T. ) ;
#10428=EDGE_CURVE ( 'NONE', #6932, #12149, #1560, .T. ) ;
#10443=DIRECTION ( 'NONE',  ( 0.3420201433256622181, -0.9396926207859107594, 0.000000000000000000 ) ) ;
#10448=ORIENTED_EDGE ( 'NONE', *, *, #17973, .T. ) ;
#10456=VERTEX_POINT ( 'NONE', #23604 ) ;
#10463=DIRECTION ( 'NONE',  ( 0.3420201433256622736, -0.9396926207859106484, -1.232595164407828100E-31 ) ) ;
#10466=CARTESIAN_POINT ( 'NONE',  ( -19.99999999999999645, -9.000000000000003553, 5.000000000000079936 ) ) ;
#10475=LINE ( 'NONE', #1324, #3838 ) ;
#10483=ORIENTED_EDGE ( 'NONE', *, *, #20431, .F. ) ;
#10484=CARTESIAN_POINT ( 'NONE',  ( 4.688305830332750723, -11.25000000000000355, 5.000000000000079936 ) ) ;
#10488=DIRECTION ( 'NONE',  ( 0.9396926207859107594, -0.3420201433256623291, 3.697785493223492838E-32 ) ) ;
#10493=PLANE ( 'NONE',  #11071 ) ;
#10506=DIRECTION ( 'NONE',  ( 0.3420201433256622181, 0.9396926207859107594, -6.162975822039141593E-32 ) ) ;
#10513=ORIENTED_EDGE ( 'NONE', *, *, #12082, .F. ) ;
#10523=CARTESIAN_POINT ( 'NONE',  ( -18.12177574676618974, -9.000000000000003553, 5.000000000000079936 ) ) ;
#10528=DIRECTION ( 'NONE',  ( 0.000000000000000000, 0.000000000000000000, -1.000000000000000000 ) ) ;
#10536=CARTESIAN_POINT ( 'NONE',  ( -1.594879469667249916, -11.25000000000000355, 5.000000000000079936 ) ) ;
#10544=FACE_OUTER_BOUND ( 'NONE', #3444, .T. ) ;
#10547=VERTEX_POINT ( 'NONE', #15120 ) ;
#10562=CARTESIAN_POINT ( 'NONE',  ( -14.98018309676618998, -9.000000000000003553, 10.00000000000008882 ) ) ;
#10564=VECTOR ( 'NONE', #21778, 1000.000000000000114 ) ;
#10565=DIRECTION ( 'NONE',  ( -6.938893903907210234E-15, 0.000000000000000000, 1.000000000000000000 ) ) ;
#10572=DIRECTION ( 'NONE',  ( 1.000000000000000000, 7.703719777548943412E-32, 0.000000000000000000 ) ) ;
#10574=CARTESIAN_POINT ( 'NONE',  ( 20.39626908033275043, -11.25000000000000355, 10.00000000000008882 ) ) ;
#10579=ORIENTED_EDGE ( 'NONE', *, *, #5696, .F. ) ;
#10594=CARTESIAN_POINT ( 'NONE',  ( 5.577176569667260608, -11.25000000000000355, 10.00000000000008882 ) ) ;
#10598=DIRECTION ( 'NONE',  ( 0.000000000000000000, 0.000000000000000000, 1.000000000000000000 ) ) ;
#10611=PLANE ( 'NONE',  #17543 ) ;
#10615=DIRECTION ( 'NONE',  ( 0.3420201433256622181, 0.9396926207859107594, -6.162975822039141593E-32 ) ) ;
#10625=ORIENTED_EDGE ( 'NONE', *, *, #22199, .T. ) ;
#10632=PLANE ( 'NONE',  #5178 ) ;
#10643=VECTOR ( 'NONE', #13659, 1000.000000000000114 ) ;
#10649=PRESENTATION_STYLE_ASSIGNMENT (( #8966 ) ) ;
#10665=EDGE_LOOP ( 'NONE', ( #1497, #22938, #21816, #21782 ) ) ;
#10669=DIRECTION ( 'NONE',  ( 0.3420201433256622181, 0.9396926207859107594, -6.162975822039141593E-32 ) ) ;
#10670=LINE ( 'NONE', #17947, #21308 ) ;
#10681=DIRECTION ( 'NONE',  ( -7.087422195345011518E-32, -1.000000000000000000, -0.000000000000000000 ) ) ;
#10686=DIRECTION ( 'NONE',  ( 0.000000000000000000, 0.000000000000000000, 1.000000000000000000 ) ) ;
#10689=CARTESIAN_POINT ( 'NONE',  ( -19.99999999999999645, -9.000000000000003553, 5.000000000000079936 ) ) ;
#10693=ORIENTED_EDGE ( 'NONE', *, *, #23667, .T. ) ;
#10694=VECTOR ( 'NONE', #796, 1000.000000000000000 ) ;
#10698=CARTESIAN_POINT ( 'NONE',  ( 21.28513981966725765, -11.25000000000000355, 10.00000000000008882 ) ) ;
#10709=VECTOR ( 'NONE', #5091, 1000.000000000000114 ) ;
#10732=AXIS2_PLACEMENT_3D ( 'NONE', #20656, #6183, #4372 ) ;
#10741=VECTOR ( 'NONE', #10847, 1000.000000000000114 ) ;
#10750=CARTESIAN_POINT ( 'NONE',  ( 23.53786173033275375, -11.25000000000000355, 5.000000000000079936 ) ) ;
#10754=DIRECTION ( 'NONE',  ( -6.779273404243054876E-32, -0.9396926207859083169, 0.3420201433256691015 ) ) ;
#10763=CARTESIAN_POINT ( 'NONE',  ( 31.59224393136097930, 9.778041110016188142, 10.00000000000008882 ) ) ;
#10772=CARTESIAN_POINT ( 'NONE',  ( 118.3095189484530181, -2.399706452296379577, 55.00000000000021316 ) ) ;
#10776=ORIENTED_EDGE ( 'NONE', *, *, #9138, .T. ) ;
#10781=VERTEX_POINT ( 'NONE', #938 ) ;
#10789=PLANE ( 'NONE',  #10347 ) ;
#10790=CARTESIAN_POINT ( 'NONE',  ( -3.847601380332740018, -11.25000000000000355, 5.000000000000079936 ) ) ;
#10792=VERTEX_POINT ( 'NONE', #21404 ) ;
#10797=CARTESIAN_POINT ( 'NONE',  ( -3.019423509283438722, -8.974600000000002353, 5.000000000000079936 ) ) ;
#10801=ORIENTED_EDGE ( 'NONE', *, *, #20765, .T. ) ;
#10805=LINE ( 'NONE', #3221, #1657 ) ;
#10807=VERTEX_POINT ( 'NONE', #10322 ) ;
#10809=CARTESIAN_POINT ( 'NONE',  ( 41.56848460323381289, -9.000000000000001776, 5.000000000000079936 ) ) ;
#10811=LINE ( 'NONE', #6831, #4389 ) ;
#10812=ORIENTED_EDGE ( 'NONE', *, *, #15246, .F. ) ;
#10847=DIRECTION ( 'NONE',  ( 0.3420201433256622181, 0.9396926207859107594, -6.162975822039141593E-32 ) ) ;
#10857=ORIENTED_EDGE ( 'NONE', *, *, #13517, .F. ) ;
#10861=DIRECTION ( 'NONE',  ( 0.9396926207859107594, -0.3420201433256623291, 3.697785493223492838E-32 ) ) ;
#10862=ORIENTED_EDGE ( 'NONE', *, *, #17156, .F. ) ;
#10868=ADVANCED_FACE ( 'NONE', ( #23204 ), #1400, .F. ) ;
#10879=CARTESIAN_POINT ( 'NONE',  ( 12.17357108409515476, 2.710222204658223610, 10.00000000000008882 ) ) ;
#10883=ORIENTED_EDGE ( 'NONE', *, *, #12316, .F. ) ;
#10887=VERTEX_POINT ( 'NONE', #19854 ) ;
#10888=LINE ( 'NONE', #23189, #7956 ) ;
#10890=ADVANCED_FACE ( 'NONE', ( #22985 ), #14139, .T. ) ;
#10892=ORIENTED_EDGE ( 'NONE', *, *, #14311, .T. ) ;
#10899=DIRECTION ( 'NONE',  ( -1.000000000000000000, -7.703719777548943412E-32, 0.000000000000000000 ) ) ;
#10901=ORIENTED_EDGE ( 'NONE', *, *, #19557, .F. ) ;
#10913=DIRECTION ( 'NONE',  ( 0.3420201433256622181, 0.9396926207859107594, -6.162975822039141593E-32 ) ) ;
#10916=PLANE ( 'NONE',  #7089 ) ;
#10917=DIRECTION ( 'NONE',  ( -7.087422195345011518E-32, -1.000000000000000000, -0.000000000000000000 ) ) ;
#10919=VECTOR ( 'NONE', #19074, 1000.000000000000000 ) ;
#10922=ORIENTED_EDGE ( 'NONE', *, *, #18195, .T. ) ;
#10927=CARTESIAN_POINT ( 'NONE',  ( 42.38741763033275589, -11.25000000000000355, 5.000000000000079936 ) ) ;
#10930=DIRECTION ( 'NONE',  ( 0.000000000000000000, 0.000000000000000000, 1.000000000000000000 ) ) ;
#10943=ORIENTED_EDGE ( 'NONE', *, *, #7622, .F. ) ;
#10949=VECTOR ( 'NONE', #7936, 1000.000000000000114 ) ;
#10964=EDGE_CURVE ( 'NONE', #3670, #18990, #12235, .T. ) ;
#10968=CARTESIAN_POINT ( 'NONE',  ( 44.70083240928345703, -8.974600000000002353, 5.000000000000079936 ) ) ;
#10973=CARTESIAN_POINT ( 'NONE',  ( 50.00000000000000000, -2.399706452296379577, 55.00000000000021316 ) ) ;
#10974=ORIENTED_EDGE ( 'NONE', *, *, #4930, .T. ) ;
#10980=CARTESIAN_POINT ( 'NONE',  ( 45.00000000000000711, -9.796556200126381952, 10.73275603335500072 ) ) ;
#10982=EDGE_CURVE ( 'NONE', #10073, #17999, #16168, .T. ) ;
#10989=EDGE_CURVE ( 'NONE', #21989, #19450, #23695, .T. ) ;
#11005=ORIENTED_EDGE ( 'NONE', *, *, #9496, .F. ) ;
#11010=DIRECTION ( 'NONE',  ( 0.000000000000000000, 5.754033390038006453E-16, 1.000000000000000000 ) ) ;
#11011=EDGE_CURVE ( 'NONE', #22026, #19360, #20198, .T. ) ;
#11012=CARTESIAN_POINT ( 'NONE',  ( 43.27628836966725601, -11.25000000000000355, 5.000000000000079936 ) ) ;
#11015=AXIS2_PLACEMENT_3D ( 'NONE', #15980, #8680, #16536 ) ;
#11016=CARTESIAN_POINT ( 'NONE',  ( 44.10446624071656174, -8.974600000000002353, 5.000000000000079936 ) ) ;
#11018=DIRECTION ( 'NONE',  ( 1.000000000000000000, 7.703719777548943412E-32, 0.000000000000000000 ) ) ;
#11029=( LENGTH_UNIT ( ) NAMED_UNIT ( * ) SI_UNIT ( .MILLI., .METRE. ) );
#11030=ORIENTED_EDGE ( 'NONE', *, *, #23089, .F. ) ;
#11031=DIRECTION ( 'NONE',  ( 0.000000000000000000, 0.000000000000000000, 1.000000000000000000 ) ) ;
#11033=CARTESIAN_POINT ( 'NONE',  ( -19.99999999999999645, -9.000000000000003553, 5.000000000000079936 ) ) ;
#11038=LINE ( 'NONE', #7794, #6827 ) ;
#11041=VECTOR ( 'NONE', #2198, 1000.000000000000114 ) ;
#11042=VECTOR ( 'NONE', #9299, 1000.000000000000114 ) ;
#11046=ADVANCED_FACE ( 'NONE', ( #3807 ), #21880, .F. ) ;
#11048=EDGE_CURVE ( 'NONE', #6771, #14744, #7313, .T. ) ;
#11056=DIRECTION ( 'NONE',  ( -7.087422195345011518E-32, -1.000000000000000000, -0.000000000000000000 ) ) ;
#11066=ORIENTED_EDGE ( 'NONE', *, *, #15741, .T. ) ;
#11067=ORIENTED_EDGE ( 'NONE', *, *, #21763, .T. ) ;
#11071=AXIS2_PLACEMENT_3D ( 'NONE', #19668, #1111, #6758 ) ;
#11078=VECTOR ( 'NONE', #15095, 1000.000000000000000 ) ;
#11090=PLANE ( 'NONE',  #4425 ) ;
#11101=VECTOR ( 'NONE', #5509, 1000.000000000000000 ) ;
#11113=DIRECTION ( 'NONE',  ( 0.000000000000000000, 0.000000000000000000, 1.000000000000000000 ) ) ;
#11115=CARTESIAN_POINT ( 'NONE',  ( 36.99310306966726358, -11.25000000000000355, 10.00000000000008882 ) ) ;
#11117=FACE_OUTER_BOUND ( 'NONE', #20485, .T. ) ;
#11119=DIRECTION ( 'NONE',  ( 0.000000000000000000, 0.000000000000000000, 1.000000000000000000 ) ) ;
#11125=ADVANCED_FACE ( 'NONE', ( #23578 ), #90, .F. ) ;
#11126=EDGE_LOOP ( 'NONE', ( #19739, #10901, #2070, #1605 ) ) ;
#11128=ORIENTED_EDGE ( 'NONE', *, *, #21666, .F. ) ;
#11129=CARTESIAN_POINT ( 'NONE',  ( -16.41397198033274307, -11.25000000000000355, 5.000000000000079936 ) ) ;
#11145=AXIS2_PLACEMENT_3D ( 'NONE', #2566, #8696, #14328 ) ;
#11151=EDGE_CURVE ( 'NONE', #4473, #19596, #12698, .T. ) ;
#11153=SURFACE_SIDE_STYLE ('',( #2004 ) ) ;
#11159=LINE ( 'NONE', #1578, #7585 ) ;
#11172=VERTEX_POINT ( 'NONE', #9581 ) ;
#11173=CARTESIAN_POINT ( 'NONE',  ( 13.29415075323382034, -9.000000000000003553, 5.000000000000079936 ) ) ;
#11180=DIRECTION ( 'NONE',  ( -1.000000000000000000, -7.703719777548943412E-32, 0.000000000000000000 ) ) ;
#11183=ORIENTED_EDGE ( 'NONE', *, *, #13944, .T. ) ;
#11189=FACE_OUTER_BOUND ( 'NONE', #21510, .T. ) ;
#11190=ORIENTED_EDGE ( 'NONE', *, *, #4733, .F. ) ;
#11193=EDGE_CURVE ( 'NONE', #10807, #10456, #11618, .T. ) ;
#11195=ADVANCED_FACE ( 'NONE', ( #4162 ), #675, .F. ) ;
#11208=ORIENTED_EDGE ( 'NONE', *, *, #9830, .F. ) ;
#11218=DIRECTION ( 'NONE',  ( -1.000000000000000000, -7.703719777548943412E-32, 0.000000000000000000 ) ) ;
#11223=EDGE_CURVE ( 'NONE', #8640, #1126, #10055, .T. ) ;
#11230=CARTESIAN_POINT ( 'NONE',  ( 44.00000000000000711, -9.796556200126378400, 10.00000000000008882 ) ) ;
#11244=AXIS2_PLACEMENT_3D ( 'NONE', #746, #20620, #2658 ) ;
#11249=ORIENTED_EDGE ( 'NONE', *, *, #7060, .F. ) ;
#11258=DIRECTION ( 'NONE',  ( 7.087422195345011518E-32, 1.000000000000000000, -0.000000000000000000 ) ) ;
#11263=SURFACE_STYLE_USAGE ( .BOTH. , #11153 ) ;
#11267=CARTESIAN_POINT ( 'NONE',  ( 40.13469571966727045, -11.25000000000000355, 5.000000000000079936 ) ) ;
#11273=DIRECTION ( 'NONE',  ( 0.000000000000000000, 0.000000000000000000, 1.000000000000000000 ) ) ;
#11284=EDGE_CURVE ( 'NONE', #14520, #12520, #7886, .T. ) ;
#11285=VECTOR ( 'NONE', #2116, 1000.000000000000114 ) ;
#11289=CARTESIAN_POINT ( 'NONE',  ( -19.99999999999999645, -15.00000000000001954, 5.000000000000079936 ) ) ;
#11300=ORIENTED_EDGE ( 'NONE', *, *, #14342, .T. ) ;
#11311=VECTOR ( 'NONE', #7260, 1000.000000000000000 ) ;
#11322=EDGE_CURVE ( 'NONE', #2408, #15944, #16225, .T. ) ;
#11326=LINE ( 'NONE', #16819, #11890 ) ;
#11329=DIRECTION ( 'NONE',  ( 0.000000000000000000, 0.000000000000000000, -1.000000000000000000 ) ) ;
#11331=ORIENTED_EDGE ( 'NONE', *, *, #10305, .F. ) ;
#11336=CARTESIAN_POINT ( 'NONE',  ( 34.67968829071656245, -8.974600000000002353, 5.000000000000079936 ) ) ;
#11337=ORIENTED_EDGE ( 'NONE', *, *, #15139, .F. ) ;
#11339=LINE ( 'NONE', #7615, #5292 ) ;
#11357=DIRECTION ( 'NONE',  ( -1.000000000000000000, -7.703719777548943412E-32, 0.000000000000000000 ) ) ;
#11364=CARTESIAN_POINT ( 'NONE',  ( 34.67044344676619971, -9.000000000000007105, 10.00000000000008882 ) ) ;
#11370=VERTEX_POINT ( 'NONE', #11413 ) ;
#11376=CARTESIAN_POINT ( 'NONE',  ( 50.00000000000000000, -10.00000000000001954, 15.00000000000002842 ) ) ;
#11392=ORIENTED_EDGE ( 'NONE', *, *, #4796, .T. ) ;
#11394=DIRECTION ( 'NONE',  ( -1.000000000000000000, -7.703719777548943412E-32, 0.000000000000000000 ) ) ;
#11397=DIRECTION ( 'NONE',  ( -0.9396926207859107594, -0.3420201433256623291, 1.540743955509804830E-32 ) ) ;
#11405=VECTOR ( 'NONE', #9351, 1000.000000000000114 ) ;
#11411=DIRECTION ( 'NONE',  ( 0.9396926207859107594, -0.3420201433256623291, 3.697785493223492838E-32 ) ) ;
#11412=AXIS2_PLACEMENT_3D ( 'NONE', #7123, #10386, #12169 ) ;
#11413=CARTESIAN_POINT ( 'NONE',  ( 15.82088754676620823, -9.000000000000005329, 5.000000000000079936 ) ) ;
#11415=DIRECTION ( 'NONE',  ( 0.000000000000000000, 0.000000000000000000, -1.000000000000000000 ) ) ;
#11421=EDGE_LOOP ( 'NONE', ( #10693, #17681, #22722, #16271 ) ) ;
#11428=ORIENTED_EDGE ( 'NONE', *, *, #4034, .F. ) ;
#11449=VERTEX_POINT ( 'NONE', #12117 ) ;
#11454=EDGE_CURVE ( 'NONE', #1550, #21989, #2627, .T. ) ;
#11456=ORIENTED_EDGE ( 'NONE', *, *, #2644, .T. ) ;
#11458=VECTOR ( 'NONE', #9718, 1000.000000000000000 ) ;
#11462=EDGE_LOOP ( 'NONE', ( #874, #13506, #18903, #18538 ) ) ;
#11481=ORIENTED_EDGE ( 'NONE', *, *, #19514, .F. ) ;
#11490=VECTOR ( 'NONE', #12961, 1000.000000000000114 ) ;
#11491=DIRECTION ( 'NONE',  ( 0.3420201433256622181, -0.9396926207859107594, 0.000000000000000000 ) ) ;
#11492=VERTEX_POINT ( 'NONE', #6594 ) ;
#11493=LINE ( 'NONE', #18766, #22132 ) ;
#11498=ADVANCED_FACE ( 'NONE', ( #17264 ), #6479, .T. ) ;
#11500=EDGE_CURVE ( 'NONE', #23556, #5711, #22509, .T. ) ;
#11509=CARTESIAN_POINT ( 'NONE',  ( 45.00000000000000000, -10.00000000000001954, 12.50000000000002665 ) ) ;
#11510=AXIS2_PLACEMENT_3D ( 'NONE', #21934, #9512, #12874 ) ;
#11514=ORIENTED_EDGE ( 'NONE', *, *, #903, .F. ) ;
#11518=ORIENTED_EDGE ( 'NONE', *, *, #18003, .F. ) ;
#11520=DIRECTION ( 'NONE',  ( 0.3420201433256622181, 0.9396926207859107594, -6.162975822039141593E-32 ) ) ;
#11524=ORIENTED_EDGE ( 'NONE', *, *, #11322, .F. ) ;
#11539=CARTESIAN_POINT ( 'NONE',  ( 37.81203609676620658, -9.000000000000005329, 5.000000000000079936 ) ) ;
#11546=EDGE_LOOP ( 'NONE', ( #1571, #22972, #10448, #688 ) ) ;
#11548=EDGE_LOOP ( 'NONE', ( #8343, #10310, #8063, #11776 ) ) ;
#11554=AXIS2_PLACEMENT_3D ( 'NONE', #15205, #4284, #4515 ) ;
#11561=PLANE ( 'NONE',  #4924 ) ;
#11571=ORIENTED_EDGE ( 'NONE', *, *, #20871, .T. ) ;
#11572=CARTESIAN_POINT ( 'NONE',  ( 45.00000000000000000, -10.00000000000001599, 34.11836509645782201 ) ) ;
#11582=EDGE_LOOP ( 'NONE', ( #6371, #21628, #19818, #23675 ) ) ;
#11589=CARTESIAN_POINT ( 'NONE',  ( -19.99999999999999645, -9.000000000000003553, 5.000000000000079936 ) ) ;
#11596=PLANE ( 'NONE',  #15702 ) ;
#11605=EDGE_CURVE ( 'NONE', #18990, #8446, #3339, .T. ) ;
#11609=ORIENTED_EDGE ( 'NONE', *, *, #22075, .T. ) ;
#11618=LINE ( 'NONE', #18887, #13463 ) ;
#11625=ADVANCED_FACE ( 'NONE', ( #6951 ), #1183, .F. ) ;
#11628=EDGE_CURVE ( 'NONE', #129, #11492, #21827, .T. ) ;
#11647=VERTEX_POINT ( 'NONE', #12599 ) ;
#11652=DIRECTION ( 'NONE',  ( 0.000000000000000000, -5.754033390038005467E-16, -1.000000000000000000 ) ) ;
#11656=PLANE ( 'NONE',  #17337 ) ;
#11680=CARTESIAN_POINT ( 'NONE',  ( 26.67945438033275707, -11.25000000000000355, 5.000000000000079936 ) ) ;
#11693=VECTOR ( 'NONE', #17101, 1000.000000000000000 ) ;
#11707=AXIS2_PLACEMENT_3D ( 'NONE', #3920, #11258, #14987 ) ;
#11724=UNCERTAINTY_MEASURE_WITH_UNIT (LENGTH_MEASURE( 1.000000000000000082E-05 ), #11029, 'distance_accuracy_value', 'NONE');
#11731=EDGE_CURVE ( 'NONE', #5149, #10094, #8747, .T. ) ;
#11733=EDGE_CURVE ( 'NONE', #20008, #21726, #23581, .T. ) ;
#11738=CARTESIAN_POINT ( 'NONE',  ( 47.85166990323382663, -9.000000000000005329, 10.00000000000008882 ) ) ;
#11740=VERTEX_POINT ( 'NONE', #18658 ) ;
#11746=LINE ( 'NONE', #23077, #23656 ) ;
#11749=CARTESIAN_POINT ( 'NONE',  ( 47.84242505928347100, -8.974600000000002353, 5.000000000000079936 ) ) ;
#11751=CARTESIAN_POINT ( 'NONE',  ( 50.00000000000000000, 15.00000000000003375, 10.00000000000008882 ) ) ;
#11755=LINE ( 'NONE', #2611, #10643 ) ;
#11757=LINE ( 'NONE', #22374, #7271 ) ;
#11771=CARTESIAN_POINT ( 'NONE',  ( -1.696909521094715823, -2.338219870597463945, 10.00000000000008882 ) ) ;
#11776=ORIENTED_EDGE ( 'NONE', *, *, #12082, .T. ) ;
#11777=AXIS2_PLACEMENT_3D ( 'NONE', #10466, #16189, #10930 ) ;
#11786=VECTOR ( 'NONE', #5704, 1000.000000000000000 ) ;
#11795=DIRECTION ( 'NONE',  ( 7.010384997569515515E-32, 1.000000000000000000, -3.469446951953615175E-16 ) ) ;
#11798=CARTESIAN_POINT ( 'NONE',  ( -19.99999999999999645, -9.000000000000003553, 5.000000000000079936 ) ) ;
#11802=AXIS2_PLACEMENT_3D ( 'NONE', #11962, #435, #15079 ) ;
#11803=ORIENTED_EDGE ( 'NONE', *, *, #3401, .F. ) ;
#11813=ORIENTED_EDGE ( 'NONE', *, *, #14552, .F. ) ;
#11829=AXIS2_PLACEMENT_3D ( 'NONE', #18180, #14614, #16044 ) ;
#11831=LINE ( 'NONE', #10270, #6637 ) ;
#11833=ORIENTED_EDGE ( 'NONE', *, *, #11868, .T. ) ;
#11842=CARTESIAN_POINT ( 'NONE',  ( -0.7060087303327398089, -11.25000000000000355, 10.00000000000008882 ) ) ;
#11844=VECTOR ( 'NONE', #21218, 1000.000000000000000 ) ;
#11849=DIRECTION ( 'NONE',  ( 1.000000000000000000, 7.703719777548943412E-32, 0.000000000000000000 ) ) ;
#11857=EDGE_LOOP ( 'NONE', ( #15782, #13038, #20817, #4416 ) ) ;
#11858=DIRECTION ( 'NONE',  ( 0.000000000000000000, 0.000000000000000000, -1.000000000000000000 ) ) ;
#11859=EDGE_CURVE ( 'NONE', #8586, #19009, #9233, .T. ) ;
#11863=ORIENTED_EDGE ( 'NONE', *, *, #19440, .F. ) ;
#11866=CARTESIAN_POINT ( 'NONE',  ( 9.546947090716562556, -8.974600000000002353, 10.00000000000008882 ) ) ;
#11868=EDGE_CURVE ( 'NONE', #21099, #22731, #21997, .T. ) ;
#11872=ORIENTED_EDGE ( 'NONE', *, *, #15305, .F. ) ;
#11890=VECTOR ( 'NONE', #397, 999.9999999999998863 ) ;
#11891=ORIENTED_EDGE ( 'NONE', *, *, #22805, .F. ) ;
#11894=DIRECTION ( 'NONE',  ( -0.3420201433256622181, 0.9396926207859106484, 1.232595164407828100E-31 ) ) ;
#11896=CARTESIAN_POINT ( 'NONE',  ( 118.3095189484530181, -2.399706452296352932, 60.00000000000021316 ) ) ;
#11899=ORIENTED_EDGE ( 'NONE', *, *, #23541, .F. ) ;
#11902=VERTEX_POINT ( 'NONE', #17236 ) ;
#11903=DIRECTION ( 'NONE',  ( 0.000000000000000000, 0.000000000000000000, -1.000000000000000000 ) ) ;
#11911=FACE_OUTER_BOUND ( 'NONE', #958, .T. ) ;
#11912=VECTOR ( 'NONE', #13917, 1000.000000000000114 ) ;
#11920=LINE ( 'NONE', #11798, #3986 ) ;
#11922=CARTESIAN_POINT ( 'NONE',  ( 28.99286915928345110, -8.974600000000002353, 5.000000000000079936 ) ) ;
#11926=ORIENTED_EDGE ( 'NONE', *, *, #20158, .T. ) ;
#11933=EDGE_LOOP ( 'NONE', ( #22729, #11481, #195, #12254 ) ) ;
#11948=CARTESIAN_POINT ( 'NONE',  ( -2.413812496766191806, -9.000000000000001776, 10.00000000000008882 ) ) ;
#11962=CARTESIAN_POINT ( 'NONE',  ( 25.85127650928345489, -8.974600000000002353, 5.000000000000079936 ) ) ;
#11969=ORIENTED_EDGE ( 'NONE', *, *, #8960, .F. ) ;
#11974=CARTESIAN_POINT ( 'NONE',  ( -9.311853653233800543, -9.000000000000005329, 10.00000000000008882 ) ) ;
#11980=EDGE_LOOP ( 'NONE', ( #13277, #10857, #16913, #8559 ) ) ;
#11988=DIRECTION ( 'NONE',  ( 0.3420201433256622736, 0.9396926207859106484, 0.000000000000000000 ) ) ;
#11990=EDGE_CURVE ( 'NONE', #5746, #9385, #20797, .T. ) ;
#11995=ORIENTED_EDGE ( 'NONE', *, *, #8808, .T. ) ;
#11998=EDGE_CURVE ( 'NONE', #313, #20062, #22961, .T. ) ;
#12015=EDGE_LOOP ( 'NONE', ( #2295, #2858, #7604, #3694 ) ) ;
#12026=DIRECTION ( 'NONE',  ( 0.000000000000000000, 0.000000000000000000, 1.000000000000000000 ) ) ;
#12027=EDGE_CURVE ( 'NONE', #13738, #7050, #22607, .T. ) ;
#12037=DIRECTION ( 'NONE',  ( 0.3420201433256622736, 0.9396926207859106484, 0.000000000000000000 ) ) ;
#12038=ORIENTED_EDGE ( 'NONE', *, *, #17584, .T. ) ;
#12041=ORIENTED_EDGE ( 'NONE', *, *, #21928, .F. ) ;
#12045=ORIENTED_EDGE ( 'NONE', *, *, #9040, .F. ) ;
#12052=CARTESIAN_POINT ( 'NONE',  ( -19.99999999999999645, -9.000000000000003553, 5.000000000000079936 ) ) ;
#12057=EDGE_CURVE ( 'NONE', #13272, #20280, #15572, .T. ) ;
#12064=EDGE_LOOP ( 'NONE', ( #20834, #13531, #23284, #10943 ) ) ;
#12068=LINE ( 'NONE', #4974, #4232 ) ;
#12075=LINE ( 'NONE', #4627, #22839 ) ;
#12076=CARTESIAN_POINT ( 'NONE',  ( 36.99310306966726358, -11.25000000000000355, 5.000000000000079936 ) ) ;
#12082=EDGE_CURVE ( 'NONE', #12965, #20008, #23553, .T. ) ;
#12090=DIRECTION ( 'NONE',  ( -0.9396926207859107594, -0.3420201433256623291, 1.540743955509804830E-32 ) ) ;
#12099=VECTOR ( 'NONE', #9312, 1000.000000000000000 ) ;
#12116=CARTESIAN_POINT ( 'NONE',  ( -12.44420145928343935, -8.974600000000002353, 5.000000000000079936 ) ) ;
#12117=CARTESIAN_POINT ( 'NONE',  ( -14.16125006966725053, -11.25000000000000355, 10.00000000000008882 ) ) ;
#12121=DIRECTION ( 'NONE',  ( 0.000000000000000000, 0.000000000000000000, -1.000000000000000000 ) ) ;
#12124=EDGE_CURVE ( 'NONE', #8828, #15755, #13885, .T. ) ;
#12138=DIRECTION ( 'NONE',  ( 0.000000000000000000, 0.000000000000000000, 1.000000000000000000 ) ) ;
#12140=VECTOR ( 'NONE', #1558, 1000.000000000000000 ) ;
#12149=VERTEX_POINT ( 'NONE', #12210 ) ;
#12158=VERTEX_POINT ( 'NONE', #2947 ) ;
#12169=DIRECTION ( 'NONE',  ( 0.000000000000000000, 0.000000000000000000, -1.000000000000000000 ) ) ;
#12178=ORIENTED_EDGE ( 'NONE', *, *, #270, .F. ) ;
#12186=ORIENTED_EDGE ( 'NONE', *, *, #17156, .T. ) ;
#12194=PLANE ( 'NONE',  #3777 ) ;
#12207=VECTOR ( 'NONE', #186, 1000.000000000000000 ) ;
#12210=CARTESIAN_POINT ( 'NONE',  ( -12.45344630323380208, -9.000000000000003553, 10.00000000000008882 ) ) ;
#12219=DIRECTION ( 'NONE',  ( 0.3420201433256622736, -0.9396926207859106484, -1.232595164407828100E-31 ) ) ;
#12222=ORIENTED_EDGE ( 'NONE', *, *, #11193, .T. ) ;
#12235=LINE ( 'NONE', #1532, #10323 ) ;
#12236=AXIS2_PLACEMENT_3D ( 'NONE', #23454, #7062, #21163 ) ;
#12239=LINE ( 'NONE', #22988, #7078 ) ;
#12246=( NAMED_UNIT ( * ) PLANE_ANGLE_UNIT ( ) SI_UNIT ( $, .RADIAN. ) );
#12247=ORIENTED_EDGE ( 'NONE', *, *, #8945, .T. ) ;
#12249=CARTESIAN_POINT ( 'NONE',  ( 8.718769219667262149, -11.25000000000000355, 10.00000000000008882 ) ) ;
#12252=VERTEX_POINT ( 'NONE', #4020 ) ;
#12254=ORIENTED_EDGE ( 'NONE', *, *, #23267, .T. ) ;
#12259=LINE ( 'NONE', #6614, #16342 ) ;
#12265=CARTESIAN_POINT ( 'NONE',  ( -19.99999999999999645, -9.000000000000003553, 5.000000000000079936 ) ) ;
#12273=ORIENTED_EDGE ( 'NONE', *, *, #15438, .F. ) ;
#12286=ORIENTED_EDGE ( 'NONE', *, *, #6410, .T. ) ;
#12293=ADVANCED_FACE ( 'NONE', ( #11117 ), #12695, .F. ) ;
#12296=AXIS2_PLACEMENT_3D ( 'NONE', #4185, #11397, #5866 ) ;
#12302=LINE ( 'NONE', #10392, #3052 ) ;
#12306=ORIENTED_EDGE ( 'NONE', *, *, #11048, .T. ) ;
#12309=ORIENTED_EDGE ( 'NONE', *, *, #4387, .F. ) ;
#12316=EDGE_CURVE ( 'NONE', #375, #3848, #7159, .T. ) ;
#12322=DIRECTION ( 'NONE',  ( -0.3420201433256622181, 0.9396926207859106484, 1.232595164407828100E-31 ) ) ;
#12326=EDGE_CURVE ( 'NONE', #6681, #12674, #20173, .T. ) ;
#12331=ORIENTED_EDGE ( 'NONE', *, *, #4364, .F. ) ;
#12337=CARTESIAN_POINT ( 'NONE',  ( 15.00195451966726523, -11.25000000000000355, 10.00000000000008882 ) ) ;
#12349=ORIENTED_EDGE ( 'NONE', *, *, #21634, .F. ) ;
#12357=CARTESIAN_POINT ( 'NONE',  ( 29.00211400323381028, -9.000000000000003553, 5.000000000000079936 ) ) ;
#12361=AXIS2_PLACEMENT_3D ( 'NONE', #2834, #460, #12573 ) ;
#12364=CARTESIAN_POINT ( 'NONE',  ( 50.00000000000000000, 10.00000000000001599, 12.50000000000002842 ) ) ;
#12368=CARTESIAN_POINT ( 'NONE',  ( 50.00000000000000000, 10.00000000000001599, 15.00000000000003020 ) ) ;
#12371=ORIENTED_EDGE ( 'NONE', *, *, #8035, .T. ) ;
#12382=DIRECTION ( 'NONE',  ( 1.000000000000000000, 7.703719777548943412E-32, 0.000000000000000000 ) ) ;
#12383=DIRECTION ( 'NONE',  ( 0.000000000000000000, 0.000000000000000000, -1.000000000000000000 ) ) ;
#12388=ORIENTED_EDGE ( 'NONE', *, *, #7237, .T. ) ;
#12403=DIRECTION ( 'NONE',  ( 0.3420201433256622181, 0.9396926207859107594, -6.162975822039141593E-32 ) ) ;
#12410=DIRECTION ( 'NONE',  ( 1.000000000000000000, 7.703719777548943412E-32, 0.000000000000000000 ) ) ;
#12421=ORIENTED_EDGE ( 'NONE', *, *, #7237, .F. ) ;
#12425=EDGE_CURVE ( 'NONE', #13738, #6569, #788, .T. ) ;
#12426=DIRECTION ( 'NONE',  ( 0.000000000000000000, 0.000000000000000000, 1.000000000000000000 ) ) ;
#12430=ORIENTED_EDGE ( 'NONE', *, *, #5031, .F. ) ;
#12438=FILL_AREA_STYLE_COLOUR ( '', #5333 ) ;
#12442=ORIENTED_EDGE ( 'NONE', *, *, #546, .T. ) ;
#12451=EDGE_LOOP ( 'NONE', ( #3134, #15522, #8059, #9239, #19224 ) ) ;
#12454=DIRECTION ( 'NONE',  ( 0.3420201433256622181, 0.9396926207859107594, -6.162975822039141593E-32 ) ) ;
#12464=DIRECTION ( 'NONE',  ( -1.000000000000000000, -7.703719777548943412E-32, 0.000000000000000000 ) ) ;
#12470=DIRECTION ( 'NONE',  ( 0.3420201433256622736, 0.9396926207859106484, 0.000000000000000000 ) ) ;
#12477=DIRECTION ( 'NONE',  ( 0.000000000000000000, 0.000000000000000000, 1.000000000000000000 ) ) ;
#12482=LINE ( 'NONE', #18078, #7265 ) ;
#12487=ADVANCED_FACE ( 'NONE', ( #13622 ), #22583, .F. ) ;
#12488=ORIENTED_EDGE ( 'NONE', *, *, #9943, .F. ) ;
#12491=VECTOR ( 'NONE', #11894, 1000.000000000000114 ) ;
#12493=ORIENTED_EDGE ( 'NONE', *, *, #7622, .T. ) ;
#12498=VECTOR ( 'NONE', #18822, 1000.000000000000000 ) ;
#12504=LINE ( 'NONE', #12265, #18743 ) ;
#12507=LINE ( 'NONE', #17988, #2639 ) ;
#12519=DIRECTION ( 'NONE',  ( 0.3420201433256622736, 0.9396926207859106484, 0.000000000000000000 ) ) ;
#12520=VERTEX_POINT ( 'NONE', #4738 ) ;
#12551=FACE_OUTER_BOUND ( 'NONE', #13809, .T. ) ;
#12552=ORIENTED_EDGE ( 'NONE', *, *, #19741, .T. ) ;
#12556=LINE ( 'NONE', #10763, #15612 ) ;
#12561=EDGE_CURVE ( 'NONE', #21784, #7680, #12068, .T. ) ;
#12570=VERTEX_POINT ( 'NONE', #19454 ) ;
#12573=DIRECTION ( 'NONE',  ( 0.000000000000000000, 0.000000000000000000, -1.000000000000000000 ) ) ;
#12577=DIRECTION ( 'NONE',  ( -3.081487911019570796E-32, -0.3420201433256691015, 0.9396926207859083169 ) ) ;
#12585=PLANE ( 'NONE',  #2268 ) ;
#12587=CARTESIAN_POINT ( 'NONE',  ( 38.41764710928345750, -8.974600000000002353, 5.000000000000079936 ) ) ;
#12590=AXIS2_PLACEMENT_3D ( 'NONE', #1839, #3640, #7142 ) ;
#12596=CARTESIAN_POINT ( 'NONE',  ( 13.28490590928345405, -8.974600000000002353, 5.000000000000079936 ) ) ;
#12599=CARTESIAN_POINT ( 'NONE',  ( -19.99999999999999645, -15.00000000000001954, 10.00000000000008882 ) ) ;
#12604=EDGE_CURVE ( 'NONE', #2044, #11740, #18384, .T. ) ;
#12606=VECTOR ( 'NONE', #12403, 1000.000000000000114 ) ;
#12614=AXIS2_PLACEMENT_3D ( 'NONE', #7904, #13540, #7792 ) ;
#12623=EDGE_CURVE ( 'NONE', #21726, #15944, #15946, .T. ) ;
#12636=VERTEX_POINT ( 'NONE', #19178 ) ;
#12643=ORIENTED_EDGE ( 'NONE', *, *, #22492, .F. ) ;
#12655=EDGE_CURVE ( 'NONE', #1035, #2408, #19524, .T. ) ;
#12664=PLANE ( 'NONE',  #20517 ) ;
#12665=FACE_OUTER_BOUND ( 'NONE', #21596, .T. ) ;
#12671=FACE_OUTER_BOUND ( 'NONE', #1026, .T. ) ;
#12674=VERTEX_POINT ( 'NONE', #9990 ) ;
#12695=PLANE ( 'NONE',  #13423 ) ;
#12696=PLANE ( 'NONE',  #23167 ) ;
#12698=CIRCLE ( 'NONE', #11554, 2.500000000000007550 ) ;
#12700=ORIENTED_EDGE ( 'NONE', *, *, #9661, .T. ) ;
#12703=VERTEX_POINT ( 'NONE', #10348 ) ;
#12712=VERTEX_POINT ( 'NONE', #1786 ) ;
#12714=FACE_OUTER_BOUND ( 'NONE', #2523, .T. ) ;
#12721=CARTESIAN_POINT ( 'NONE',  ( -19.99999999999999645, -9.000000000000003553, 5.000000000000079936 ) ) ;
#12723=CARTESIAN_POINT ( 'NONE',  ( -14.16125006966725053, -11.25000000000000355, 5.000000000000079936 ) ) ;
#12727=CARTESIAN_POINT ( 'NONE',  ( 43.27628836966725601, -11.25000000000000355, 5.000000000000079936 ) ) ;
#12728=LINE ( 'NONE', #3583, #5157 ) ;
#12743=DIRECTION ( 'NONE',  ( 7.087422195345011518E-32, 1.000000000000000000, -0.000000000000000000 ) ) ;
#12755=ORIENTED_EDGE ( 'NONE', *, *, #10128, .F. ) ;
#12772=VERTEX_POINT ( 'NONE', #10927 ) ;
#12773=DIRECTION ( 'NONE',  ( -7.087422195345011518E-32, -1.000000000000000000, -0.000000000000000000 ) ) ;
#12782=CARTESIAN_POINT ( 'NONE',  ( 2.435583919667260400, -11.25000000000000355, 5.000000000000079936 ) ) ;
#12790=VECTOR ( 'NONE', #3767, 1000.000000000000000 ) ;
#12792=VECTOR ( 'NONE', #9117, 1000.000000000000114 ) ;
#12797=CARTESIAN_POINT ( 'NONE',  ( 45.00000000000000000, -10.00000000000001954, 17.50000000000002842 ) ) ;
#12798=LINE ( 'NONE', #23431, #17042 ) ;
#12809=LINE ( 'NONE', #7298, #7243 ) ;
#12810=ORIENTED_EDGE ( 'NONE', *, *, #11990, .T. ) ;
#12820=DIRECTION ( 'NONE',  ( -1.000000000000000000, -7.703719777548943412E-32, 0.000000000000000000 ) ) ;
#12826=ORIENTED_EDGE ( 'NONE', *, *, #8960, .T. ) ;
#12835=VECTOR ( 'NONE', #17955, 1000.000000000000114 ) ;
#12836=ORIENTED_EDGE ( 'NONE', *, *, #18852, .F. ) ;
#12853=DIRECTION ( 'NONE',  ( -7.087422195345011518E-32, -1.000000000000000000, -0.000000000000000000 ) ) ;
#12865=ORIENTED_EDGE ( 'NONE', *, *, #11151, .F. ) ;
#12866=VECTOR ( 'NONE', #9653, 1000.000000000000114 ) ;
#12868=VECTOR ( 'NONE', #4402, 1000.000000000000000 ) ;
#12874=DIRECTION ( 'NONE',  ( -1.000000000000000000, -7.703719777548943412E-32, 0.000000000000000000 ) ) ;
#12881=DIRECTION ( 'NONE',  ( 0.000000000000000000, 0.000000000000000000, -1.000000000000000000 ) ) ;
#12895=CARTESIAN_POINT ( 'NONE',  ( -18.12177574676618974, -9.000000000000003553, 5.000000000000079936 ) ) ;
#12908=DIRECTION ( 'NONE',  ( 7.087422195345011518E-32, 1.000000000000000000, 0.000000000000000000 ) ) ;
#12916=ORIENTED_EDGE ( 'NONE', *, *, #19741, .F. ) ;
#12921=VERTEX_POINT ( 'NONE', #22012 ) ;
#12926=DIRECTION ( 'NONE',  ( -0.3420201433256622181, 0.9396926207859106484, 1.232595164407828100E-31 ) ) ;
#12928=CARTESIAN_POINT ( 'NONE',  ( 45.00000000000000000, -15.00000000000001954, 11.00000000000008882 ) ) ;
#12929=ORIENTED_EDGE ( 'NONE', *, *, #7030, .F. ) ;
#12937=CARTESIAN_POINT ( 'NONE',  ( 39.91453229447491680, 12.80710635516961382, 10.00000000000008882 ) ) ;
#12940=EDGE_LOOP ( 'NONE', ( #5386, #14159, #7169, #16553 ) ) ;
#12951=CARTESIAN_POINT ( 'NONE',  ( -6.989194030332740226, -11.25000000000000355, 5.000000000000079936 ) ) ;
#12961=DIRECTION ( 'NONE',  ( 0.3420201433256622181, -0.9396926207859107594, 0.000000000000000000 ) ) ;
#12965=VERTEX_POINT ( 'NONE', #109 ) ;
#12975=CARTESIAN_POINT ( 'NONE',  ( 50.38765154071656838, -8.974600000000002353, 10.00000000000008882 ) ) ;
#13015=VECTOR ( 'NONE', #1122, 1000.000000000000000 ) ;
#13016=LINE ( 'NONE', #7498, #18676 ) ;
#13018=ADVANCED_FACE ( 'NONE', ( #7909 ), #13080, .F. ) ;
#13019=CARTESIAN_POINT ( 'NONE',  ( -19.99999999999999645, -9.000000000000003553, 10.00000000000008882 ) ) ;
#13025=ADVANCED_FACE ( 'NONE', ( #9713 ), #18800, .F. ) ;
#13027=CARTESIAN_POINT ( 'NONE',  ( -19.99999999999999645, -9.000000000000003553, 10.00000000000008882 ) ) ;
#13036=DIRECTION ( 'NONE',  ( 0.9396926207859107594, -0.3420201433256623291, 3.697785493223492838E-32 ) ) ;
#13037=PLANE ( 'NONE',  #13596 ) ;
#13038=ORIENTED_EDGE ( 'NONE', *, *, #9394, .F. ) ;
#13043=ORIENTED_EDGE ( 'NONE', *, *, #753, .F. ) ;
#13044=DIRECTION ( 'NONE',  ( 0.3420201433256622181, -0.9396926207859107594, 0.000000000000000000 ) ) ;
#13045=ORIENTED_EDGE ( 'NONE', *, *, #13752, .F. ) ;
#13074=ORIENTED_EDGE ( 'NONE', *, *, #3401, .T. ) ;
#13077=CARTESIAN_POINT ( 'NONE',  ( 118.3095189484530181, 10.00000000000001599, 15.00000000000003020 ) ) ;
#13078=EDGE_CURVE ( 'NONE', #2784, #16998, #472, .T. ) ;
#13080=PLANE ( 'NONE',  #20266 ) ;
#13082=PLANE ( 'NONE',  #4190 ) ;
#13086=ORIENTED_EDGE ( 'NONE', *, *, #1544, .F. ) ;
#13088=DIRECTION ( 'NONE',  ( 0.000000000000000000, 5.754033390038004481E-16, -1.000000000000000000 ) ) ;
#13112=EDGE_CURVE ( 'NONE', #5198, #10249, #19146, .T. ) ;
#13119=CARTESIAN_POINT ( 'NONE',  ( 49.55947366966726264, -11.25000000000000355, 10.00000000000008882 ) ) ;
#13121=CARTESIAN_POINT ( 'NONE',  ( 33.85151041966726382, -11.25000000000000355, 5.000000000000079936 ) ) ;
#13128=VECTOR ( 'NONE', #20564, 1000.000000000000000 ) ;
#13135=DIRECTION ( 'NONE',  ( -4.930380657631312836E-32, -0.3420201433256691015, -0.9396926207859083169 ) ) ;
#13145=EDGE_CURVE ( 'NONE', #20787, #12636, #6694, .T. ) ;
#13149=DIRECTION ( 'NONE',  ( 0.000000000000000000, 0.000000000000000000, 1.000000000000000000 ) ) ;
#13156=ORIENTED_EDGE ( 'NONE', *, *, #15013, .T. ) ;
#13157=LINE ( 'NONE', #902, #10694 ) ;
#13158=EDGE_LOOP ( 'NONE', ( #1421, #15171, #3676, #12421 ) ) ;
#13164=CARTESIAN_POINT ( 'NONE',  ( 9.546947090716562556, -8.974600000000002353, 5.000000000000079936 ) ) ;
#13165=EDGE_LOOP ( 'NONE', ( #14665, #896, #7635, #5261 ) ) ;
#13177=ADVANCED_FACE ( 'NONE', ( #5097 ), #23419, .F. ) ;
#13181=ORIENTED_EDGE ( 'NONE', *, *, #21829, .T. ) ;
#13186=LINE ( 'NONE', #7109, #17893 ) ;
#13194=FACE_OUTER_BOUND ( 'NONE', #6952, .T. ) ;
#13196=ORIENTED_EDGE ( 'NONE', *, *, #2620, .F. ) ;
#13198=VECTOR ( 'NONE', #13475, 1000.000000000000114 ) ;
#13209=LINE ( 'NONE', #11896, #10371 ) ;
#13216=EDGE_CURVE ( 'NONE', #3172, #16212, #17917, .T. ) ;
#13221=VERTEX_POINT ( 'NONE', #10410 ) ;
#13240=VERTEX_POINT ( 'NONE', #10523 ) ;
#13250=EDGE_CURVE ( 'NONE', #6771, #1981, #12556, .T. ) ;
#13251=CARTESIAN_POINT ( 'NONE',  ( 36.99310306966726358, -11.25000000000000355, 5.000000000000079936 ) ) ;
#13254=VECTOR ( 'NONE', #2375, 1000.000000000000000 ) ;
#13272=VERTEX_POINT ( 'NONE', #16361 ) ;
#13276=CARTESIAN_POINT ( 'NONE',  ( -13.27237933033274153, -11.25000000000000355, 10.00000000000008882 ) ) ;
#13277=ORIENTED_EDGE ( 'NONE', *, *, #22492, .T. ) ;
#13283=DIRECTION ( 'NONE',  ( 1.000000000000000000, 7.703719777548943412E-32, 0.000000000000000000 ) ) ;
#13296=VECTOR ( 'NONE', #17746, 1000.000000000000000 ) ;
#13297=EDGE_LOOP ( 'NONE', ( #12836, #21480, #3018, #8118 ) ) ;
#13298=DIRECTION ( 'NONE',  ( 0.000000000000000000, 0.000000000000000000, 1.000000000000000000 ) ) ;
#13299=CARTESIAN_POINT ( 'NONE',  ( 23.53786173033275375, -11.25000000000000355, 5.000000000000079936 ) ) ;
#13317=CARTESIAN_POINT ( 'NONE',  ( 48.67060293033276963, -11.25000000000000355, 10.00000000000008882 ) ) ;
#13325=LINE ( 'NONE', #20594, #8648 ) ;
#13329=CIRCLE ( 'NONE', #19406, 2.500000000000007550 ) ;
#13339=VECTOR ( 'NONE', #9656, 1000.000000000000000 ) ;
#13346=VECTOR ( 'NONE', #22887, 1000.000000000000000 ) ;
#13351=FACE_OUTER_BOUND ( 'NONE', #4300, .T. ) ;
#13355=CARTESIAN_POINT ( 'NONE',  ( 46.41788101966725577, -11.25000000000000355, 10.00000000000008882 ) ) ;
#13380=DIRECTION ( 'NONE',  ( 0.3420201433256622181, 0.9396926207859107594, -6.162975822039141593E-32 ) ) ;
#13387=LINE ( 'NONE', #9783, #3428 ) ;
#13406=EDGE_CURVE ( 'NONE', #4376, #15000, #20754, .T. ) ;
#13412=DIRECTION ( 'NONE',  ( -0.3420201433256622181, 0.9396926207859106484, 1.232595164407828100E-31 ) ) ;
#13422=FACE_OUTER_BOUND ( 'NONE', #23345, .T. ) ;
#13423=AXIS2_PLACEMENT_3D ( 'NONE', #7402, #7636, #14959 ) ;
#13447=CARTESIAN_POINT ( 'NONE',  ( 118.3095189484530181, 15.00000000000003375, 34.11836509645780069 ) ) ;
#13448=DIRECTION ( 'NONE',  ( 1.000000000000000000, 7.703719777548943412E-32, 0.000000000000000000 ) ) ;
#13451=CARTESIAN_POINT ( 'NONE',  ( 44.71007725323381976, -9.000000000000000000, 5.000000000000079936 ) ) ;
#13456=ORIENTED_EDGE ( 'NONE', *, *, #1502, .T. ) ;
#13462=EDGE_LOOP ( 'NONE', ( #4293, #13625 ) ) ;
#13463=VECTOR ( 'NONE', #17099, 1000.000000000000000 ) ;
#13466=ADVANCED_FACE ( 'NONE', ( #8924 ), #1110, .T. ) ;
#13475=DIRECTION ( 'NONE',  ( -0.3420201433256622181, 0.9396926207859106484, 1.232595164407828100E-31 ) ) ;
#13477=CARTESIAN_POINT ( 'NONE',  ( -19.99999999999999645, -9.000000000000003553, 10.00000000000008882 ) ) ;
#13489=CARTESIAN_POINT ( 'NONE',  ( 23.26995556824705602, 6.748975864862779339, 10.00000000000008882 ) ) ;
#13490=ORIENTED_EDGE ( 'NONE', *, *, #15548, .F. ) ;
#13491=ADVANCED_FACE ( 'NONE', ( #19667 ), #8563, .F. ) ;
#13506=ORIENTED_EDGE ( 'NONE', *, *, #2371, .T. ) ;
#13509=EDGE_CURVE ( 'NONE', #15051, #15217, #1225, .T. ) ;
#13511=ORIENTED_EDGE ( 'NONE', *, *, #18009, .T. ) ;
#13513=CARTESIAN_POINT ( 'NONE',  ( 41.56848460323381289, -9.000000000000003553, 5.000000000000079936 ) ) ;
#13515=ORIENTED_EDGE ( 'NONE', *, *, #5529, .F. ) ;
#13517=EDGE_CURVE ( 'NONE', #19575, #13757, #6876, .T. ) ;
#13520=ORIENTED_EDGE ( 'NONE', *, *, #5073, .F. ) ;
#13526=DIRECTION ( 'NONE',  ( 0.3420201433256622736, -0.9396926207859106484, -1.232595164407828100E-31 ) ) ;
#13527=ORIENTED_EDGE ( 'NONE', *, *, #18112, .F. ) ;
#13531=ORIENTED_EDGE ( 'NONE', *, *, #17394, .F. ) ;
#13533=FACE_OUTER_BOUND ( 'NONE', #2959, .T. ) ;
#13535=DIRECTION ( 'NONE',  ( 0.000000000000000000, 0.000000000000000000, 1.000000000000000000 ) ) ;
#13540=DIRECTION ( 'NONE',  ( 1.000000000000000000, 7.703719777548943412E-32, 0.000000000000000000 ) ) ;
#13544=DIRECTION ( 'NONE',  ( 0.000000000000000000, 0.000000000000000000, -1.000000000000000000 ) ) ;
#13549=ORIENTED_EDGE ( 'NONE', *, *, #21288, .T. ) ;
#13557=VERTEX_POINT ( 'NONE', #17542 ) ;
#13563=VERTEX_POINT ( 'NONE', #3389 ) ;
#13572=CARTESIAN_POINT ( 'NONE',  ( 0.7277801532338084023, -9.000000000000003553, 5.000000000000079936 ) ) ;
#13582=CARTESIAN_POINT ( 'NONE',  ( 38.42689195323381313, -9.000000000000001776, 10.00000000000008882 ) ) ;
#13584=DIRECTION ( 'NONE',  ( 0.3420201433256622181, -0.9396926207859107594, 0.000000000000000000 ) ) ;
#13587=LINE ( 'NONE', #13477, #22575 ) ;
#13588=ORIENTED_EDGE ( 'NONE', *, *, #21634, .T. ) ;
#13589=FACE_BOUND ( 'NONE', #16238, .T. ) ;
#13596=AXIS2_PLACEMENT_3D ( 'NONE', #16608, #187, #7518 ) ;
#13608=CARTESIAN_POINT ( 'NONE',  ( 12.68853974071656232, -8.974600000000002353, 10.00000000000008882 ) ) ;
#13619=DIRECTION ( 'NONE',  ( 0.000000000000000000, 0.000000000000000000, -1.000000000000000000 ) ) ;
#13622=FACE_OUTER_BOUND ( 'NONE', #6854, .T. ) ;
#13625=ORIENTED_EDGE ( 'NONE', *, *, #15236, .T. ) ;
#13632=AXIS2_PLACEMENT_3D ( 'NONE', #915, #12090, #13993 ) ;
#13636=ORIENTED_EDGE ( 'NONE', *, *, #11868, .F. ) ;
#13637=CARTESIAN_POINT ( 'NONE',  ( -3.847601380332740018, -11.25000000000000355, 5.000000000000079936 ) ) ;
#13641=DIRECTION ( 'NONE',  ( 0.000000000000000000, 0.000000000000000000, 1.000000000000000000 ) ) ;
#13645=ORIENTED_EDGE ( 'NONE', *, *, #585, .T. ) ;
#13649=ORIENTED_EDGE ( 'NONE', *, *, #4072, .F. ) ;
#13650=CARTESIAN_POINT ( 'NONE',  ( 16.43574340323381122, -9.000000000000003553, 5.000000000000079936 ) ) ;
#13652=CARTESIAN_POINT ( 'NONE',  ( 45.00000000000000000, -10.00000000000001599, 34.11836509645782201 ) ) ;
#13658=PLANE ( 'NONE',  #23650 ) ;
#13659=DIRECTION ( 'NONE',  ( 0.3420201433256622181, -0.9396926207859107594, 0.000000000000000000 ) ) ;
#13669=EDGE_CURVE ( 'NONE', #8446, #17296, #2139, .T. ) ;
#13675=ORIENTED_EDGE ( 'NONE', *, *, #20801, .T. ) ;
#13677=DIRECTION ( 'NONE',  ( 0.000000000000000000, 0.000000000000000000, 1.000000000000000000 ) ) ;
#13678=CARTESIAN_POINT ( 'NONE',  ( 0.7277801532338118440, -9.000000000000003553, 10.00000000000008882 ) ) ;
#13694=CARTESIAN_POINT ( 'NONE',  ( 22.70968385928345157, -8.974600000000002353, 5.000000000000079936 ) ) ;
#13697=CARTESIAN_POINT ( 'NONE',  ( 11.86036186966726191, -11.25000000000000355, 10.00000000000008882 ) ) ;
#13715=ADVANCED_FACE ( 'NONE', ( #16899 ), #353, .F. ) ;
#13723=DIRECTION ( 'NONE',  ( -7.087422195345011518E-32, -1.000000000000000000, -0.000000000000000000 ) ) ;
#13724=VECTOR ( 'NONE', #1134, 1000.000000000000000 ) ;
#13728=LINE ( 'NONE', #9775, #9341 ) ;
#13735=AXIS2_PLACEMENT_3D ( 'NONE', #3149, #17665, #19318 ) ;
#13738=VERTEX_POINT ( 'NONE', #15116 ) ;
#13742=ORIENTED_EDGE ( 'NONE', *, *, #5031, .T. ) ;
#13744=ADVANCED_FACE ( 'NONE', ( #5986 ), #20582, .F. ) ;
#13748=DIRECTION ( 'NONE',  ( -0.3420201433256622181, 0.9396926207859106484, 1.232595164407828100E-31 ) ) ;
#13752=EDGE_CURVE ( 'NONE', #20363, #20481, #4120, .T. ) ;
#13757=VERTEX_POINT ( 'NONE', #934 ) ;
#13764=CARTESIAN_POINT ( 'NONE',  ( -8.696997796766188671, -9.000000000000003553, 5.000000000000079936 ) ) ;
#13765=DIRECTION ( 'NONE',  ( 0.000000000000000000, 0.000000000000000000, -1.000000000000000000 ) ) ;
#13767=CARTESIAN_POINT ( 'NONE',  ( -2.423057340716551433, -8.974600000000002353, 5.000000000000079936 ) ) ;
#13775=FACE_OUTER_BOUND ( 'NONE', #1687, .T. ) ;
#13789=DIRECTION ( 'NONE',  ( 1.000000000000000000, 7.703719777548943412E-32, 0.000000000000000000 ) ) ;
#13794=VECTOR ( 'NONE', #21372, 1000.000000000000114 ) ;
#13805=LINE ( 'NONE', #15723, #7013 ) ;
#13807=VERTEX_POINT ( 'NONE', #13900 ) ;
#13808=LINE ( 'NONE', #4321, #944 ) ;
#13809=EDGE_LOOP ( 'NONE', ( #12038, #380, #86, #16880 ) ) ;
#13825=DIRECTION ( 'NONE',  ( 0.3420201433256622181, -0.9396926207859107594, 0.000000000000000000 ) ) ;
#13830=CARTESIAN_POINT ( 'NONE',  ( 10.14331325928345073, -8.974600000000002353, 5.000000000000079936 ) ) ;
#13840=VERTEX_POINT ( 'NONE', #8157 ) ;
#13852=DIRECTION ( 'NONE',  ( 0.000000000000000000, 0.000000000000000000, 1.000000000000000000 ) ) ;
#13861=DIRECTION ( 'NONE',  ( 0.3420201433256622181, 0.9396926207859107594, -6.162975822039141593E-32 ) ) ;
#13863=ORIENTED_EDGE ( 'NONE', *, *, #2528, .F. ) ;
#13867=ORIENTED_EDGE ( 'NONE', *, *, #4387, .T. ) ;
#13868=CARTESIAN_POINT ( 'NONE',  ( 22.11331769071655984, -8.974600000000002353, 10.00000000000008882 ) ) ;
#13876=ORIENTED_EDGE ( 'NONE', *, *, #8691, .T. ) ;
#13885=LINE ( 'NONE', #17813, #15716 ) ;
#13888=EDGE_CURVE ( 'NONE', #11740, #2044, #13329, .T. ) ;
#13890=LINE ( 'NONE', #11866, #19433 ) ;
#13894=CARTESIAN_POINT ( 'NONE',  ( -19.99999999999999645, -11.25000000000000355, 10.00000000000008882 ) ) ;
#13895=ORIENTED_EDGE ( 'NONE', *, *, #5397, .T. ) ;
#13899=CARTESIAN_POINT ( 'NONE',  ( -19.99999999999999645, -9.000000000000003553, 5.000000000000079936 ) ) ;
#13900=CARTESIAN_POINT ( 'NONE',  ( 3.254516946766202512, -9.000000000000001776, 10.00000000000008882 ) ) ;
#13909=CARTESIAN_POINT ( 'NONE',  ( 45.52901028033275566, -11.25000000000000355, 5.000000000000079936 ) ) ;
#13917=DIRECTION ( 'NONE',  ( -0.3420201433256622181, 0.9396926207859106484, 1.232595164407828100E-31 ) ) ;
#13927=ORIENTED_EDGE ( 'NONE', *, *, #16782, .F. ) ;
#13931=DIRECTION ( 'NONE',  ( 0.3420201433256622181, 0.9396926207859107594, -6.162975822039141593E-32 ) ) ;
#13932=EDGE_CURVE ( 'NONE', #23556, #6771, #17254, .T. ) ;
#13935=EDGE_CURVE ( 'NONE', #4844, #19360, #23333, .T. ) ;
#13939=CARTESIAN_POINT ( 'NONE',  ( 10.15255810323380992, -9.000000000000001776, 5.000000000000079936 ) ) ;
#13942=CARTESIAN_POINT ( 'NONE',  ( 50.00000000000000000, -15.00000000000003375, 34.11836509645780779 ) ) ;
#13944=EDGE_CURVE ( 'NONE', #20363, #6074, #18294, .T. ) ;
#13945=EDGE_LOOP ( 'NONE', ( #23623, #8123, #6625, #16616 ) ) ;
#13970=EDGE_CURVE ( 'NONE', #12520, #23136, #14494, .T. ) ;
#13976=VECTOR ( 'NONE', #17206, 1000.000000000000000 ) ;
#13978=VECTOR ( 'NONE', #23208, 1000.000000000000114 ) ;
#13983=FACE_OUTER_BOUND ( 'NONE', #2724, .T. ) ;
#13986=CIRCLE ( 'NONE', #21983, 2.500000000000007550 ) ;
#13993=DIRECTION ( 'NONE',  ( 0.3420201433256622736, -0.9396926207859106484, -1.232595164407828100E-31 ) ) ;
#14004=DIRECTION ( 'NONE',  ( -0.9396926207859107594, -0.3420201433256623291, 1.540743955509804830E-32 ) ) ;
#14007=ORIENTED_EDGE ( 'NONE', *, *, #22075, .F. ) ;
#14008=ADVANCED_FACE ( 'NONE', ( #16043 ), #7055, .F. ) ;
#14011=DIRECTION ( 'NONE',  ( 0.000000000000000000, 0.000000000000000000, 1.000000000000000000 ) ) ;
#14022=LINE ( 'NONE', #4907, #7026 ) ;
#14041=DIRECTION ( 'NONE',  ( -1.000000000000000000, -7.703719777548943412E-32, 0.000000000000000000 ) ) ;
#14048=LINE ( 'NONE', #19893, #6895 ) ;
#14049=ORIENTED_EDGE ( 'NONE', *, *, #15142, .T. ) ;
#14056=CARTESIAN_POINT ( 'NONE',  ( 50.00000000000000000, 2.399706452296353820, 60.00000000000021316 ) ) ;
#14061=EDGE_CURVE ( 'NONE', #14828, #5147, #10670, .T. ) ;
#14071=EDGE_CURVE ( 'NONE', #20787, #7410, #3564, .T. ) ;
#14077=CARTESIAN_POINT ( 'NONE',  ( 17.25467643033275067, -11.25000000000000355, 5.000000000000079936 ) ) ;
#14098=VECTOR ( 'NONE', #19341, 1000.000000000000000 ) ;
#14102=ADVANCED_FACE ( 'NONE', ( #20674 ), #6075, .F. ) ;
#14104=EDGE_CURVE ( 'NONE', #18482, #21534, #21987, .T. ) ;
#14106=EDGE_CURVE ( 'NONE', #14872, #4634, #1989, .T. ) ;
#14110=CARTESIAN_POINT ( 'NONE',  ( 28.39650299071657003, -8.974600000000002353, 5.000000000000079936 ) ) ;
#14115=AXIS2_PLACEMENT_3D ( 'NONE', #17115, #8258, #22612 ) ;
#14117=ORIENTED_EDGE ( 'NONE', *, *, #17317, .T. ) ;
#14125=CARTESIAN_POINT ( 'NONE',  ( 19.57733605323380743, -9.000000000000001776, 5.000000000000079936 ) ) ;
#14129=VECTOR ( 'NONE', #6877, 1000.000000000000000 ) ;
#14134=DIRECTION ( 'NONE',  ( -1.000000000000000000, -7.703719777548943412E-32, 0.000000000000000000 ) ) ;
#14139=PLANE ( 'NONE',  #12236 ) ;
#14159=ORIENTED_EDGE ( 'NONE', *, *, #9138, .F. ) ;
#14168=LINE ( 'NONE', #14286, #16719 ) ;
#14170=VECTOR ( 'NONE', #2337, 1000.000000000000000 ) ;
#14191=VECTOR ( 'NONE', #19412, 1000.000000000000114 ) ;
#14194=ORIENTED_EDGE ( 'NONE', *, *, #11628, .F. ) ;
#14202=VECTOR ( 'NONE', #23511, 1000.000000000000000 ) ;
#14218=LINE ( 'NONE', #5085, #11311 ) ;
#14222=FACE_OUTER_BOUND ( 'NONE', #458, .T. ) ;
#14225=CARTESIAN_POINT ( 'NONE',  ( 42.38741763033275589, -11.25000000000000355, 10.00000000000008882 ) ) ;
#14226=AXIS2_PLACEMENT_3D ( 'NONE', #22469, #20902, #2714 ) ;
#14233=LINE ( 'NONE', #16140, #15693 ) ;
#14242=DIRECTION ( 'NONE',  ( 0.000000000000000000, 0.000000000000000000, -1.000000000000000000 ) ) ;
#14243=DIRECTION ( 'NONE',  ( 0.3420201433256622736, -0.9396926207859106484, -1.232595164407828100E-31 ) ) ;
#14248=LINE ( 'NONE', #1386, #6860 ) ;
#14259=ORIENTED_EDGE ( 'NONE', *, *, #7202, .T. ) ;
#14267=ORIENTED_EDGE ( 'NONE', *, *, #1202, .T. ) ;
#14286=CARTESIAN_POINT ( 'NONE',  ( 42.38741763033275589, -11.25000000000000355, 5.000000000000079936 ) ) ;
#14289=LINE ( 'NONE', #14410, #9161 ) ;
#14311=EDGE_CURVE ( 'NONE', #21477, #11647, #1669, .T. ) ;
#14315=DIRECTION ( 'NONE',  ( 7.087422195345011518E-32, 1.000000000000000000, -0.000000000000000000 ) ) ;
#14328=DIRECTION ( 'NONE',  ( 2.465190328815655597E-32, 0.3420201433256690460, -0.9396926207859082059 ) ) ;
#14330=CARTESIAN_POINT ( 'NONE',  ( -14.98018309676619175, -9.000000000000003553, 5.000000000000079936 ) ) ;
#14333=ORIENTED_EDGE ( 'NONE', *, *, #21731, .F. ) ;
#14342=EDGE_CURVE ( 'NONE', #11449, #17388, #5150, .T. ) ;
#14349=DIRECTION ( 'NONE',  ( 7.087422195345011518E-32, 1.000000000000000000, -0.000000000000000000 ) ) ;
#14370=AXIS2_PLACEMENT_3D ( 'NONE', #10689, #17963, #10214 ) ;
#14372=VECTOR ( 'NONE', #8492, 1000.000000000000000 ) ;
#14375=CARTESIAN_POINT ( 'NONE',  ( -19.99999999999999645, -9.000000000000003553, 10.00000000000008882 ) ) ;
#14379=EDGE_CURVE ( 'NONE', #14967, #21785, #470, .T. ) ;
#14384=DIRECTION ( 'NONE',  ( 0.9396926207859107594, -0.3420201433256623291, 3.697785493223492838E-32 ) ) ;
#14385=ORIENTED_EDGE ( 'NONE', *, *, #10989, .F. ) ;
#14390=ORIENTED_EDGE ( 'NONE', *, *, #13970, .T. ) ;
#14393=LINE ( 'NONE', #1547, #20045 ) ;
#14394=ORIENTED_EDGE ( 'NONE', *, *, #5899, .F. ) ;
#14396=ORIENTED_EDGE ( 'NONE', *, *, #23602, .T. ) ;
#14403=CARTESIAN_POINT ( 'NONE',  ( 47.85166990323382663, -9.000000000000003553, 5.000000000000079936 ) ) ;
#14404=EDGE_CURVE ( 'NONE', #21785, #12149, #11038, .T. ) ;
#14410=CARTESIAN_POINT ( 'NONE',  ( 22.10407284676620066, -9.000000000000003553, 5.000000000000079936 ) ) ;
#14417=DIRECTION ( 'NONE',  ( 0.000000000000000000, 0.000000000000000000, 1.000000000000000000 ) ) ;
#14420=VERTEX_POINT ( 'NONE', #14754 ) ;
#14425=ORIENTED_EDGE ( 'NONE', *, *, #21928, .T. ) ;
#14429=ORIENTED_EDGE ( 'NONE', *, *, #19440, .T. ) ;
#14434=LINE ( 'NONE', #16336, #10741 ) ;
#14438=CARTESIAN_POINT ( 'NONE',  ( -19.99999999999999645, -9.000000000000003553, 10.00000000000008882 ) ) ;
#14441=VECTOR ( 'NONE', #13135, 1000.000000000000000 ) ;
#14443=ORIENTED_EDGE ( 'NONE', *, *, #15013, .F. ) ;
#14446=VERTEX_POINT ( 'NONE', #20098 ) ;
#14460=DIRECTION ( 'NONE',  ( -0.3420201433256622181, 0.9396926207859106484, 1.232595164407828100E-31 ) ) ;
#14462=VECTOR ( 'NONE', #692, 1000.000000000000000 ) ;
#14465=FACE_OUTER_BOUND ( 'NONE', #16475, .T. ) ;
#14477=DIRECTION ( 'NONE',  ( 0.000000000000000000, 0.000000000000000000, -1.000000000000000000 ) ) ;
#14488=ORIENTED_EDGE ( 'NONE', *, *, #639, .T. ) ;
#14491=VECTOR ( 'NONE', #4536, 1000.000000000000000 ) ;
#14492=LINE ( 'NONE', #9097, #9193 ) ;
#14494=LINE ( 'NONE', #14375, #2200 ) ;
#14499=LINE ( 'NONE', #23693, #19469 ) ;
#14508=EDGE_CURVE ( 'NONE', #549, #5170, #16646, .T. ) ;
#14510=LINE ( 'NONE', #4052, #20388 ) ;
#14514=CARTESIAN_POINT ( 'NONE',  ( 34.67968829071656245, -8.974600000000002353, 10.00000000000008882 ) ) ;
#14515=FACE_OUTER_BOUND ( 'NONE', #15911, .T. ) ;
#14517=ADVANCED_FACE ( 'NONE', ( #7552 ), #5749, .F. ) ;
#14520=VERTEX_POINT ( 'NONE', #2135 ) ;
#14523=AXIS2_PLACEMENT_3D ( 'NONE', #11751, #2607, #9950 ) ;
#14551=ORIENTED_EDGE ( 'NONE', *, *, #13145, .T. ) ;
#14552=EDGE_CURVE ( 'NONE', #15223, #21477, #10192, .T. ) ;
#14567=LINE ( 'NONE', #5078, #4333 ) ;
#14570=ORIENTED_EDGE ( 'NONE', *, *, #23156, .F. ) ;
#14575=AXIS2_PLACEMENT_3D ( 'NONE', #5168, #7100, #10598 ) ;
#14579=ORIENTED_EDGE ( 'NONE', *, *, #6862, .F. ) ;
#14582=CARTESIAN_POINT ( 'NONE',  ( 45.52901028033275566, -11.25000000000000355, 10.00000000000008882 ) ) ;
#14591=DIRECTION ( 'NONE',  ( 1.000000000000000000, 7.703719777548943412E-32, 0.000000000000000000 ) ) ;
#14592=FACE_OUTER_BOUND ( 'NONE', #17342, .T. ) ;
#14600=FACE_OUTER_BOUND ( 'NONE', #15545, .T. ) ;
#14601=ORIENTED_EDGE ( 'NONE', *, *, #22231, .T. ) ;
#14606=ORIENTED_EDGE ( 'NONE', *, *, #5523, .F. ) ;
#14607=CARTESIAN_POINT ( 'NONE',  ( 118.3095189484530181, 15.00000000000003375, 34.11836509645780069 ) ) ;
#14611=ADVANCED_FACE ( 'NONE', ( #8507 ), #13658, .F. ) ;
#14614=DIRECTION ( 'NONE',  ( 0.9396926207859107594, -0.3420201433256623291, 3.697785493223492838E-32 ) ) ;
#14624=ORIENTED_EDGE ( 'NONE', *, *, #4944, .F. ) ;
#14644=ORIENTED_EDGE ( 'NONE', *, *, #16539, .T. ) ;
#14646=VECTOR ( 'NONE', #2481, 1000.000000000000000 ) ;
#14658=ORIENTED_EDGE ( 'NONE', *, *, #4864, .T. ) ;
#14662=CARTESIAN_POINT ( 'NONE',  ( 45.00000000000000000, 10.00000000000001599, 34.11836509645782201 ) ) ;
#14664=EDGE_CURVE ( 'NONE', #7460, #19492, #4803, .T. ) ;
#14665=ORIENTED_EDGE ( 'NONE', *, *, #22563, .T. ) ;
#14669=EDGE_CURVE ( 'NONE', #20897, #23413, #966, .T. ) ;
#14684=CARTESIAN_POINT ( 'NONE',  ( 44.09522139676619901, -9.000000000000003553, 5.000000000000079936 ) ) ;
#14690=FACE_OUTER_BOUND ( 'NONE', #1193, .T. ) ;
#14698=LINE ( 'NONE', #3761, #7563 ) ;
#14700=CIRCLE ( 'NONE', #22704, 5.000000000000011546 ) ;
#14703=FACE_OUTER_BOUND ( 'NONE', #18105, .T. ) ;
#14715=CARTESIAN_POINT ( 'NONE',  ( -4.736472119667250347, -11.25000000000000355, 5.000000000000079936 ) ) ;
#14717=VERTEX_POINT ( 'NONE', #9135 ) ;
#14728=DIRECTION ( 'NONE',  ( 0.3420201433256622736, 0.9396926207859106484, 0.000000000000000000 ) ) ;
#14732=CARTESIAN_POINT ( 'NONE',  ( 45.00000000000000000, -15.00000000000003375, 34.11836509645780779 ) ) ;
#14742=( LENGTH_UNIT ( ) NAMED_UNIT ( * ) SI_UNIT ( .MILLI., .METRE. ) );
#14744=VERTEX_POINT ( 'NONE', #18091 ) ;
#14745=EDGE_CURVE ( 'NONE', #20280, #20897, #14759, .T. ) ;
#14754=CARTESIAN_POINT ( 'NONE',  ( 21.28513981966725765, -11.25000000000000355, 5.000000000000079936 ) ) ;
#14756=CARTESIAN_POINT ( 'NONE',  ( 2.435583919667260400, -11.25000000000000355, 5.000000000000079936 ) ) ;
#14759=LINE ( 'NONE', #3591, #17162 ) ;
#14761=AXIS2_PLACEMENT_3D ( 'NONE', #16061, #6715, #2866 ) ;
#14768=CARTESIAN_POINT ( 'NONE',  ( 33.85151041966726382, -11.25000000000000355, 5.000000000000079936 ) ) ;
#14772=LINE ( 'NONE', #12975, #19509 ) ;
#14787=AXIS2_PLACEMENT_3D ( 'NONE', #13767, #23069, #13526 ) ;
#14794=CARTESIAN_POINT ( 'NONE',  ( 29.00211400323381028, -9.000000000000005329, 10.00000000000008882 ) ) ;
#14801=VERTEX_POINT ( 'NONE', #21901 ) ;
#14812=CARTESIAN_POINT ( 'NONE',  ( 18.14354716966726144, -11.25000000000000355, 5.000000000000079936 ) ) ;
#14816=EDGE_CURVE ( 'NONE', #18435, #12712, #16507, .T. ) ;
#14828=VERTEX_POINT ( 'NONE', #7180 ) ;
#14831=ADVANCED_FACE ( 'NONE', ( #20075 ), #16164, .F. ) ;
#14836=ADVANCED_FACE ( 'NONE', ( #1646 ), #5243, .F. ) ;
#14854=DIRECTION ( 'NONE',  ( -7.087422195345011518E-32, -1.000000000000000000, -0.000000000000000000 ) ) ;
#14872=VERTEX_POINT ( 'NONE', #11012 ) ;
#14874=DIRECTION ( 'NONE',  ( 0.3420201433256622181, 0.9396926207859107594, -6.162975822039141593E-32 ) ) ;
#14879=CYLINDRICAL_SURFACE ( 'NONE', #19855, 5.000000000000011546 ) ;
#14884=LINE ( 'NONE', #11173, #714 ) ;
#14902=DIRECTION ( 'NONE',  ( 0.3420201433256622181, -0.9396926207859107594, 0.000000000000000000 ) ) ;
#14912=VECTOR ( 'NONE', #21721, 1000.000000000000000 ) ;
#14914=CARTESIAN_POINT ( 'NONE',  ( -18.72738675928344065, -8.974600000000002353, 5.000000000000079936 ) ) ;
#14933=DIRECTION ( 'NONE',  ( 0.000000000000000000, -5.754033390038003495E-16, 1.000000000000000000 ) ) ;
#14938=CARTESIAN_POINT ( 'NONE',  ( -19.99999999999999645, -9.000000000000003553, 5.000000000000079936 ) ) ;
#14939=EDGE_LOOP ( 'NONE', ( #6944, #2840, #23653, #7739, #12186, #21717, #19744, #9378, #22633, #7903, #13549, #1327 ) ) ;
#14942=AXIS2_PLACEMENT_3D ( 'NONE', #5574, #14349, #7278 ) ;
#14948=DIRECTION ( 'NONE',  ( 1.000000000000000000, 7.703719777548943412E-32, 0.000000000000000000 ) ) ;
#14954=PLANE ( 'NONE',  #10732 ) ;
#14959=DIRECTION ( 'NONE',  ( 0.3420201433256622736, 0.9396926207859106484, 0.000000000000000000 ) ) ;
#14960=LINE ( 'NONE', #4021, #21723 ) ;
#14963=ORIENTED_EDGE ( 'NONE', *, *, #11454, .T. ) ;
#14967=VERTEX_POINT ( 'NONE', #3565 ) ;
#14983=CARTESIAN_POINT ( 'NONE',  ( 44.00000000000000711, -15.00000000000001954, 11.00000000000008882 ) ) ;
#14985=FACE_OUTER_BOUND ( 'NONE', #3167, .T. ) ;
#14987=DIRECTION ( 'NONE',  ( 0.000000000000000000, 0.000000000000000000, 1.000000000000000000 ) ) ;
#14992=CARTESIAN_POINT ( 'NONE',  ( 18.97172504071656363, -8.974600000000002353, 5.000000000000079936 ) ) ;
#14994=DIRECTION ( 'NONE',  ( 0.000000000000000000, 0.000000000000000000, 1.000000000000000000 ) ) ;
#14996=DIRECTION ( 'NONE',  ( -1.000000000000000000, -7.703719777548943412E-32, 0.000000000000000000 ) ) ;
#15000=VERTEX_POINT ( 'NONE', #12928 ) ;
#15005=DIRECTION ( 'NONE',  ( 0.9396926207859107594, -0.3420201433256623291, 3.697785493223492838E-32 ) ) ;
#15013=EDGE_CURVE ( 'NONE', #22188, #16763, #6287, .T. ) ;
#15026=ORIENTED_EDGE ( 'NONE', *, *, #1001, .T. ) ;
#15051=VERTEX_POINT ( 'NONE', #16952 ) ;
#15060=VECTOR ( 'NONE', #11180, 1000.000000000000000 ) ;
#15075=ORIENTED_EDGE ( 'NONE', *, *, #7365, .F. ) ;
#15079=DIRECTION ( 'NONE',  ( 0.3420201433256622736, -0.9396926207859106484, -1.232595164407828100E-31 ) ) ;
#15092=LINE ( 'NONE', #18885, #9545 ) ;
#15095=DIRECTION ( 'NONE',  ( 0.000000000000000000, 0.000000000000000000, 1.000000000000000000 ) ) ;
#15099=VERTEX_POINT ( 'NONE', #18745 ) ;
#15100=DIRECTION ( 'NONE',  ( -1.000000000000000000, -7.703719777548943412E-32, 0.000000000000000000 ) ) ;
#15102=ORIENTED_EDGE ( 'NONE', *, *, #19737, .T. ) ;
#15108=VERTEX_POINT ( 'NONE', #20755 ) ;
#15116=CARTESIAN_POINT ( 'NONE',  ( 3.869372803233808611, -9.000000000000001776, 5.000000000000079936 ) ) ;
#15120=CARTESIAN_POINT ( 'NONE',  ( 2.435583919667260400, -11.25000000000000355, 10.00000000000008882 ) ) ;
#15127=DIRECTION ( 'NONE',  ( -1.000000000000000000, -7.703719777548943412E-32, 0.000000000000000000 ) ) ;
#15137=PLANE ( 'NONE',  #15534 ) ;
#15139=EDGE_CURVE ( 'NONE', #16212, #2919, #21104, .T. ) ;
#15142=EDGE_CURVE ( 'NONE', #17845, #2131, #3390, .T. ) ;
#15145=VECTOR ( 'NONE', #6487, 1000.000000000000000 ) ;
#15158=LINE ( 'NONE', #22778, #10919 ) ;
#15171=ORIENTED_EDGE ( 'NONE', *, *, #13250, .F. ) ;
#15190=ORIENTED_EDGE ( 'NONE', *, *, #8560, .F. ) ;
#15205=CARTESIAN_POINT ( 'NONE',  ( 50.00000000000000000, 10.00000000000001599, 15.00000000000003020 ) ) ;
#15207=DIRECTION ( 'NONE',  ( 1.000000000000000000, 7.703719777548943412E-32, 0.000000000000000000 ) ) ;
#15213=DIRECTION ( 'NONE',  ( 1.000000000000000000, 7.703719777548943412E-32, 0.000000000000000000 ) ) ;
#15217=VERTEX_POINT ( 'NONE', #8809 ) ;
#15220=FACE_OUTER_BOUND ( 'NONE', #12064, .T. ) ;
#15223=VERTEX_POINT ( 'NONE', #23269 ) ;
#15224=CARTESIAN_POINT ( 'NONE',  ( -13.27237933033274153, -11.25000000000000355, 5.000000000000079936 ) ) ;
#15230=DIRECTION ( 'NONE',  ( 0.9396926207859107594, -0.3420201433256623291, 3.697785493223492838E-32 ) ) ;
#15233=AXIS2_PLACEMENT_3D ( 'NONE', #23191, #14004, #12219 ) ;
#15234=ADVANCED_FACE ( 'NONE', ( #2907 ), #23391, .T. ) ;
#15236=EDGE_CURVE ( 'NONE', #4233, #22239, #22122, .T. ) ;
#15243=LINE ( 'NONE', #6121, #15060 ) ;
#15246=EDGE_CURVE ( 'NONE', #13807, #12252, #6995, .T. ) ;
#15247=ADVANCED_FACE ( 'NONE', ( #23035 ), #10493, .F. ) ;
#15249=CARTESIAN_POINT ( 'NONE',  ( 20.39626908033275043, -11.25000000000000355, 5.000000000000079936 ) ) ;
#15250=ORIENTED_EDGE ( 'NONE', *, *, #14404, .T. ) ;
#15257=AXIS2_PLACEMENT_3D ( 'NONE', #6283, #7847, #4003 ) ;
#15270=FACE_OUTER_BOUND ( 'NONE', #22810, .T. ) ;
#15275=LINE ( 'NONE', #1948, #19884 ) ;
#15289=ORIENTED_EDGE ( 'NONE', *, *, #5858, .T. ) ;
#15292=CIRCLE ( 'NONE', #12614, 5.000000000000011546 ) ;
#15294=AXIS2_PLACEMENT_3D ( 'NONE', #14983, #1768, #16875 ) ;
#15298=CARTESIAN_POINT ( 'NONE',  ( -14.98018309676618998, -9.000000000000003553, 5.000000000000079936 ) ) ;
#15305=EDGE_CURVE ( 'NONE', #18254, #6932, #20103, .T. ) ;
#15320=CARTESIAN_POINT ( 'NONE',  ( 12.67929489676620314, -9.000000000000005329, 5.000000000000079936 ) ) ;
#15322=CARTESIAN_POINT ( 'NONE',  ( 44.06356521511867896, -9.086974644262722833, 10.00151577544548509 ) ) ;
#15334=DIRECTION ( 'NONE',  ( 0.000000000000000000, 0.000000000000000000, -1.000000000000000000 ) ) ;
#15338=CARTESIAN_POINT ( 'NONE',  ( -10.13078668033273999, -11.25000000000000355, 5.000000000000079936 ) ) ;
#15339=PLANE ( 'NONE',  #1220 ) ;
#15350=EDGE_CURVE ( 'NONE', #10073, #4715, #14884, .T. ) ;
#15354=FACE_OUTER_BOUND ( 'NONE', #7583, .T. ) ;
#15359=VECTOR ( 'NONE', #17744, 1000.000000000000000 ) ;
#15365=CARTESIAN_POINT ( 'NONE',  ( -19.99999999999999645, -9.000000000000003553, 5.000000000000079936 ) ) ;
#15370=CARTESIAN_POINT ( 'NONE',  ( 39.24582498033275613, -11.25000000000000355, 5.000000000000079936 ) ) ;
#15373=ORIENTED_EDGE ( 'NONE', *, *, #2461, .F. ) ;
#15379=ORIENTED_EDGE ( 'NONE', *, *, #3832, .F. ) ;
#15383=VERTEX_POINT ( 'NONE', #13317 ) ;
#15388=EDGE_CURVE ( 'NONE', #15720, #15000, #22379, .T. ) ;
#15396=CARTESIAN_POINT ( 'NONE',  ( 27.56832511966726784, -11.25000000000000355, 5.000000000000079936 ) ) ;
#15398=DIRECTION ( 'NONE',  ( 1.000000000000000000, 7.703719777548943412E-32, 0.000000000000000000 ) ) ;
#15399=ORIENTED_EDGE ( 'NONE', *, *, #20000, .F. ) ;
#15426=CYLINDRICAL_SURFACE ( 'NONE', #6254, 1.000000000000002665 ) ;
#15432=ORIENTED_EDGE ( 'NONE', *, *, #15861, .T. ) ;
#15438=EDGE_CURVE ( 'NONE', #21630, #7680, #9611, .T. ) ;
#15452=DIRECTION ( 'NONE',  ( 0.000000000000000000, 0.000000000000000000, -1.000000000000000000 ) ) ;
#15454=ORIENTED_EDGE ( 'NONE', *, *, #22334, .T. ) ;
#15455=VECTOR ( 'NONE', #18856, 1000.000000000000000 ) ;
#15456=DIRECTION ( 'NONE',  ( -1.000000000000000000, -7.703719777548943412E-32, 0.000000000000000000 ) ) ;
#15459=CARTESIAN_POINT ( 'NONE',  ( -19.99999999999999645, -9.000000000000003553, 5.000000000000079936 ) ) ;
#15460=ORIENTED_EDGE ( 'NONE', *, *, #17642, .T. ) ;
#15466=LINE ( 'NONE', #10196, #8792 ) ;
#15467=CARTESIAN_POINT ( 'NONE',  ( 39.24582498033275613, -11.25000000000000355, 5.000000000000079936 ) ) ;
#15469=ORIENTED_EDGE ( 'NONE', *, *, #12057, .T. ) ;
#15480=FACE_OUTER_BOUND ( 'NONE', #16087, .T. ) ;
#15489=ORIENTED_EDGE ( 'NONE', *, *, #6100, .T. ) ;
#15490=CARTESIAN_POINT ( 'NONE',  ( 32.96263968033274949, -11.25000000000000355, 5.000000000000079936 ) ) ;
#15492=ORIENTED_EDGE ( 'NONE', *, *, #23101, .F. ) ;
#15494=VECTOR ( 'NONE', #13584, 1000.000000000000114 ) ;
#15498=VECTOR ( 'NONE', #4111, 1000.000000000000114 ) ;
#15500=DIRECTION ( 'NONE',  ( -0.9396926207859107594, -0.3420201433256623291, 1.540743955509804830E-32 ) ) ;
#15503=EDGE_CURVE ( 'NONE', #9402, #21784, #828, .T. ) ;
#15522=ORIENTED_EDGE ( 'NONE', *, *, #15865, .F. ) ;
#15523=AXIS2_PLACEMENT_3D ( 'NONE', #4075, #11411, #9724 ) ;
#15534=AXIS2_PLACEMENT_3D ( 'NONE', #7357, #9498, #134 ) ;
#15545=EDGE_LOOP ( 'NONE', ( #13045, #11183, #22425, #19334 ) ) ;
#15548=EDGE_CURVE ( 'NONE', #19360, #5511, #19374, .T. ) ;
#15550=VECTOR ( 'NONE', #14996, 1000.000000000000000 ) ;
#15552=ORIENTED_EDGE ( 'NONE', *, *, #8623, .F. ) ;
#15553=AXIS2_PLACEMENT_3D ( 'NONE', #15338, #8141, #15452 ) ;
#15571=ORIENTED_EDGE ( 'NONE', *, *, #17861, .T. ) ;
#15572=LINE ( 'NONE', #22836, #9219 ) ;
#15574=CARTESIAN_POINT ( 'NONE',  ( -15.59503895323380362, -9.000000000000003553, 5.000000000000079936 ) ) ;
#15575=LINE ( 'NONE', #22838, #15790 ) ;
#15578=PLANE ( 'NONE',  #18941 ) ;
#15584=ORIENTED_EDGE ( 'NONE', *, *, #23089, .T. ) ;
#15585=CARTESIAN_POINT ( 'NONE',  ( -18.72738675928344065, -8.974600000000002353, 5.000000000000079936 ) ) ;
#15595=CARTESIAN_POINT ( 'NONE',  ( 25.24566549676620397, -9.000000000000001776, 5.000000000000079936 ) ) ;
#15596=VECTOR ( 'NONE', #7389, 1000.000000000000000 ) ;
#15600=CARTESIAN_POINT ( 'NONE',  ( -16.41397198033274307, -11.25000000000000355, 5.000000000000079936 ) ) ;
#15609=EDGE_LOOP ( 'NONE', ( #12810, #18966, #4445, #23410 ) ) ;
#15612=VECTOR ( 'NONE', #14460, 1000.000000000000114 ) ;
#15626=DIRECTION ( 'NONE',  ( -1.000000000000000000, -7.703719777548943412E-32, 0.000000000000000000 ) ) ;
#15631=FACE_OUTER_BOUND ( 'NONE', #3410, .T. ) ;
#15657=CARTESIAN_POINT ( 'NONE',  ( 15.00195451966726523, -11.25000000000000355, 5.000000000000079936 ) ) ;
#15660=CARTESIAN_POINT ( 'NONE',  ( 50.00000000000000000, -14.82704866393690857, 20.85615788968264894 ) ) ;
#15668=CYLINDRICAL_SURFACE ( 'NONE', #306, 2.500000000000009326 ) ;
#15679=ORIENTED_EDGE ( 'NONE', *, *, #8976, .F. ) ;
#15690=LINE ( 'NONE', #18896, #18571 ) ;
#15693=VECTOR ( 'NONE', #21490, 1000.000000000000000 ) ;
#15694=FACE_OUTER_BOUND ( 'NONE', #21748, .T. ) ;
#15699=CARTESIAN_POINT ( 'NONE',  ( -9.302608809283439584, -8.974600000000002353, 10.00000000000008882 ) ) ;
#15702=AXIS2_PLACEMENT_3D ( 'NONE', #3892, #16847, #7860 ) ;
#15705=DIRECTION ( 'NONE',  ( 0.000000000000000000, 0.000000000000000000, -1.000000000000000000 ) ) ;
#15711=VECTOR ( 'NONE', #4483, 1000.000000000000000 ) ;
#15716=VECTOR ( 'NONE', #21257, 1000.000000000000000 ) ;
#15720=VERTEX_POINT ( 'NONE', #14732 ) ;
#15722=DIRECTION ( 'NONE',  ( -1.000000000000000000, -7.703719777548943412E-32, 0.000000000000000000 ) ) ;
#15723=CARTESIAN_POINT ( 'NONE',  ( 118.3095189484530181, 15.00000000000001954, 10.00000000000008882 ) ) ;
#15725=VERTEX_POINT ( 'NONE', #1993 ) ;
#15732=ORIENTED_EDGE ( 'NONE', *, *, #6439, .F. ) ;
#15733=ORIENTED_EDGE ( 'NONE', *, *, #16451, .T. ) ;
#15737=CARTESIAN_POINT ( 'NONE',  ( -19.99999999999999645, -15.00000000000001954, 5.000000000000079936 ) ) ;
#15741=EDGE_CURVE ( 'NONE', #4177, #6681, #5485, .T. ) ;
#15750=ORIENTED_EDGE ( 'NONE', *, *, #13406, .T. ) ;
#15751=CARTESIAN_POINT ( 'NONE',  ( 31.52885079676620705, -9.000000000000005329, 10.00000000000008882 ) ) ;
#15755=VERTEX_POINT ( 'NONE', #17950 ) ;
#15772=DIRECTION ( 'NONE',  ( 0.000000000000000000, 0.000000000000000000, 1.000000000000000000 ) ) ;
#15774=EDGE_CURVE ( 'NONE', #2729, #19492, #14499, .T. ) ;
#15782=ORIENTED_EDGE ( 'NONE', *, *, #2229, .T. ) ;
#15783=CARTESIAN_POINT ( 'NONE',  ( 36.99310306966726358, -11.25000000000000355, 10.00000000000008882 ) ) ;
#15785=ORIENTED_EDGE ( 'NONE', *, *, #22805, .T. ) ;
#15787=UNCERTAINTY_MEASURE_WITH_UNIT (LENGTH_MEASURE( 1.000000000000000082E-05 ), #16369, 'distance_accuracy_value', 'NONE');
#15790=VECTOR ( 'NONE', #6452, 1000.000000000000000 ) ;
#15800=DIRECTION ( 'NONE',  ( 0.000000000000000000, 0.000000000000000000, 1.000000000000000000 ) ) ;
#15801=EDGE_CURVE ( 'NONE', #15108, #15051, #21641, .T. ) ;
#15807=LINE ( 'NONE', #5118, #1811 ) ;
#15808=ORIENTED_EDGE ( 'NONE', *, *, #21664, .T. ) ;
#15814=CARTESIAN_POINT ( 'NONE',  ( 50.00000000000000000, 2.399706452296379577, 55.00000000000021316 ) ) ;
#15823=DIRECTION ( 'NONE',  ( 0.3420201433256622736, 0.9396926207859106484, 0.000000000000000000 ) ) ;
#15824=ORIENTED_EDGE ( 'NONE', *, *, #20956, .F. ) ;
#15826=ADVANCED_FACE ( 'NONE', ( #12714 ), #18184, .T. ) ;
#15828=DIRECTION ( 'NONE',  ( 0.3420201433256622181, 0.9396926207859107594, -6.162975822039141593E-32 ) ) ;
#15830=ORIENTED_EDGE ( 'NONE', *, *, #4095, .F. ) ;
#15838=ORIENTED_EDGE ( 'NONE', *, *, #1502, .F. ) ;
#15843=VECTOR ( 'NONE', #4365, 1000.000000000000114 ) ;
#15861=EDGE_CURVE ( 'NONE', #17500, #5746, #18069, .T. ) ;
#15865=EDGE_CURVE ( 'NONE', #14872, #633, #16512, .T. ) ;
#15872=DIRECTION ( 'NONE',  ( 0.000000000000000000, 0.000000000000000000, 1.000000000000000000 ) ) ;
#15884=ORIENTED_EDGE ( 'NONE', *, *, #5585, .F. ) ;
#15889=ORIENTED_EDGE ( 'NONE', *, *, #17288, .F. ) ;
#15892=CARTESIAN_POINT ( 'NONE',  ( 38.42689195323381313, -9.000000000000003553, 5.000000000000079936 ) ) ;
#15897=AXIS2_PLACEMENT_3D ( 'NONE', #689, #8022, #14994 ) ;
#15899=VECTOR ( 'NONE', #5845, 1000.000000000000000 ) ;
#15911=EDGE_LOOP ( 'NONE', ( #1211, #21357, #7499, #1685 ) ) ;
#15920=VECTOR ( 'NONE', #15722, 1000.000000000000000 ) ;
#15941=DIRECTION ( 'NONE',  ( 0.000000000000000000, 0.000000000000000000, 1.000000000000000000 ) ) ;
#15944=VERTEX_POINT ( 'NONE', #2113 ) ;
#15946=LINE ( 'NONE', #3122, #5005 ) ;
#15954=EDGE_CURVE ( 'NONE', #19596, #11740, #9690, .T. ) ;
#15973=LINE ( 'NONE', #10370, #9132 ) ;
#15975=FACE_OUTER_BOUND ( 'NONE', #15609, .T. ) ;
#15976=EDGE_LOOP ( 'NONE', ( #1827, #19117, #22960, #13645 ) ) ;
#15980=CARTESIAN_POINT ( 'NONE',  ( -19.99999999999999645, -9.000000000000003553, 5.000000000000079936 ) ) ;
#15981=AXIS2_PLACEMENT_3D ( 'NONE', #2385, #15230, #17011 ) ;
#16008=DIRECTION ( 'NONE',  ( -1.000000000000000000, -7.703719777548943412E-32, 0.000000000000000000 ) ) ;
#16009=VECTOR ( 'NONE', #12426, 1000.000000000000000 ) ;
#16023=FACE_OUTER_BOUND ( 'NONE', #11857, .T. ) ;
#16024=VECTOR ( 'NONE', #17707, 1000.000000000000000 ) ;
#16030=PLANE ( 'NONE',  #7470 ) ;
#16033=CARTESIAN_POINT ( 'NONE',  ( 16.43574340323381122, -9.000000000000001776, 10.00000000000008882 ) ) ;
#16034=VECTOR ( 'NONE', #23236, 1000.000000000000000 ) ;
#16038=EDGE_LOOP ( 'NONE', ( #19309, #13636, #15571, #16863 ) ) ;
#16043=FACE_OUTER_BOUND ( 'NONE', #5411, .T. ) ;
#16044=DIRECTION ( 'NONE',  ( 0.3420201433256622736, 0.9396926207859106484, 0.000000000000000000 ) ) ;
#16045=ORIENTED_EDGE ( 'NONE', *, *, #3169, .F. ) ;
#16049=AXIS2_PLACEMENT_3D ( 'NONE', #13899, #2735, #6812 ) ;
#16055=ORIENTED_EDGE ( 'NONE', *, *, #877, .T. ) ;
#16061=CARTESIAN_POINT ( 'NONE',  ( 15.83013239071656741, -8.974600000000002353, 5.000000000000079936 ) ) ;
#16086=DIRECTION ( 'NONE',  ( 1.000000000000000000, 7.703719777548943412E-32, 0.000000000000000000 ) ) ;
#16087=EDGE_LOOP ( 'NONE', ( #15373, #15785, #8090, #22824 ) ) ;
#16088=EDGE_CURVE ( 'NONE', #8446, #19331, #15092, .T. ) ;
#16098=CARTESIAN_POINT ( 'NONE',  ( -10.13078668033273999, -11.25000000000000355, 5.000000000000079936 ) ) ;
#16111=AXIS2_PLACEMENT_3D ( 'NONE', #5255, #10681, #10565 ) ;
#16120=ORIENTED_EDGE ( 'NONE', *, *, #17080, .F. ) ;
#16132=CARTESIAN_POINT ( 'NONE',  ( -19.99999999999999645, -9.000000000000003553, 5.000000000000079936 ) ) ;
#16134=EDGE_CURVE ( 'NONE', #14520, #17845, #20900, .T. ) ;
#16140=CARTESIAN_POINT ( 'NONE',  ( 36.10423233033275636, -11.25000000000000355, 5.000000000000079936 ) ) ;
#16152=EDGE_CURVE ( 'NONE', #23005, #22090, #6789, .T. ) ;
#16163=DIRECTION ( 'NONE',  ( -7.087422195345011518E-32, -1.000000000000000000, -0.000000000000000000 ) ) ;
#16164=PLANE ( 'NONE',  #11829 ) ;
#16168=LINE ( 'NONE', #12596, #19079 ) ;
#16182=CARTESIAN_POINT ( 'NONE',  ( 0.1129242967662022479, -9.000000000000001776, 5.000000000000079936 ) ) ;
#16183=ORIENTED_EDGE ( 'NONE', *, *, #7742, .F. ) ;
#16189=DIRECTION ( 'NONE',  ( 7.087422195345011518E-32, 1.000000000000000000, -0.000000000000000000 ) ) ;
#16190=ADVANCED_FACE ( 'NONE', ( #2826 ), #17464, .F. ) ;
#16212=VERTEX_POINT ( 'NONE', #13637 ) ;
#16225=LINE ( 'NONE', #14438, #14202 ) ;
#16231=DIRECTION ( 'NONE',  ( 7.087422195345011518E-32, 1.000000000000000000, -0.000000000000000000 ) ) ;
#16238=EDGE_LOOP ( 'NONE', ( #16357, #17994, #8504, #11833 ) ) ;
#16240=VECTOR ( 'NONE', #19471, 1000.000000000000000 ) ;
#16241=PLANE ( 'NONE',  #12590 ) ;
#16257=( NAMED_UNIT ( * ) PLANE_ANGLE_UNIT ( ) SI_UNIT ( $, .RADIAN. ) );
#16259=LINE ( 'NONE', #23548, #17803 ) ;
#16271=ORIENTED_EDGE ( 'NONE', *, *, #17458, .T. ) ;
#16277=DIRECTION ( 'NONE',  ( 0.9396926207859107594, -0.3420201433256623291, 3.697785493223492838E-32 ) ) ;
#16279=ADVANCED_FACE ( 'NONE', ( #14465 ), #7393, .T. ) ;
#16283=CARTESIAN_POINT ( 'NONE',  ( 45.00000000000000000, 15.00000000000001954, 10.00000000000008882 ) ) ;
#16305=VECTOR ( 'NONE', #13149, 1000.000000000000000 ) ;
#16318=PLANE ( 'NONE',  #11707 ) ;
#16336=CARTESIAN_POINT ( 'NONE',  ( 6.405354440716562792, -8.974600000000002353, 5.000000000000079936 ) ) ;
#16342=VECTOR ( 'NONE', #13931, 1000.000000000000114 ) ;
#16343=VERTEX_POINT ( 'NONE', #18265 ) ;
#16344=DIRECTION ( 'NONE',  ( 1.000000000000000000, 7.703719777548943412E-32, 0.000000000000000000 ) ) ;
#16350=DIRECTION ( 'NONE',  ( -4.930380657631312836E-32, -0.3420201433256691015, -0.9396926207859083169 ) ) ;
#16354=ADVANCED_FACE ( 'NONE', ( #14592 ), #5343, .F. ) ;
#16357=ORIENTED_EDGE ( 'NONE', *, *, #19256, .T. ) ;
#16361=CARTESIAN_POINT ( 'NONE',  ( 7.829898480332751376, -11.25000000000000355, 10.00000000000008882 ) ) ;
#16369=( LENGTH_UNIT ( ) NAMED_UNIT ( * ) SI_UNIT ( .MILLI., .METRE. ) );
#16378=VECTOR ( 'NONE', #2546, 1000.000000000000000 ) ;
#16401=CARTESIAN_POINT ( 'NONE',  ( 8.718769219667262149, -11.25000000000000355, 5.000000000000079936 ) ) ;
#16407=VECTOR ( 'NONE', #13825, 1000.000000000000114 ) ;
#16420=EDGE_CURVE ( 'NONE', #5838, #2784, #14233, .T. ) ;
#16429=DIRECTION ( 'NONE',  ( 0.000000000000000000, 0.000000000000000000, 1.000000000000000000 ) ) ;
#16433=CARTESIAN_POINT ( 'NONE',  ( -0.7060087303327398089, -11.25000000000000355, 5.000000000000079936 ) ) ;
#16435=CARTESIAN_POINT ( 'NONE',  ( 49.55947366966726264, -11.25000000000000355, 5.000000000000079936 ) ) ;
#16451=EDGE_CURVE ( 'NONE', #23288, #10547, #2207, .T. ) ;
#16472=EDGE_LOOP ( 'NONE', ( #23649, #19050, #8606, #1956 ) ) ;
#16475=EDGE_LOOP ( 'NONE', ( #7375, #13588, #20121, #20536 ) ) ;
#16479=VECTOR ( 'NONE', #4419, 1000.000000000000114 ) ;
#16489=DIRECTION ( 'NONE',  ( -1.000000000000000000, -7.703719777548943412E-32, 0.000000000000000000 ) ) ;
#16492=ORIENTED_EDGE ( 'NONE', *, *, #19256, .F. ) ;
#16495=DIRECTION ( 'NONE',  ( -1.000000000000000000, -7.703719777548943412E-32, 0.000000000000000000 ) ) ;
#16496=VECTOR ( 'NONE', #13448, 1000.000000000000000 ) ;
#16507=LINE ( 'NONE', #7418, #8754 ) ;
#16512=LINE ( 'NONE', #11016, #357 ) ;
#16517=CARTESIAN_POINT ( 'NONE',  ( -3.019423509283438722, -8.974600000000002353, 10.00000000000008882 ) ) ;
#16522=CARTESIAN_POINT ( 'NONE',  ( 44.00000000000000711, -15.00000000000001954, 10.00000000000008882 ) ) ;
#16526=DIRECTION ( 'NONE',  ( 0.000000000000000000, 0.000000000000000000, -1.000000000000000000 ) ) ;
#16527=LINE ( 'NONE', #18900, #22049 ) ;
#16531=ORIENTED_EDGE ( 'NONE', *, *, #23679, .T. ) ;
#16536=DIRECTION ( 'NONE',  ( 0.000000000000000000, 0.000000000000000000, 1.000000000000000000 ) ) ;
#16539=EDGE_CURVE ( 'NONE', #13221, #3801, #5692, .T. ) ;
#16546=DIRECTION ( 'NONE',  ( -1.000000000000000000, -7.703719777548943412E-32, 0.000000000000000000 ) ) ;
#16548=FACE_OUTER_BOUND ( 'NONE', #842, .T. ) ;
#16551=EDGE_CURVE ( 'NONE', #6074, #6488, #7273, .T. ) ;
#16553=ORIENTED_EDGE ( 'NONE', *, *, #4864, .F. ) ;
#16559=VERTEX_POINT ( 'NONE', #2444 ) ;
#16579=ORIENTED_EDGE ( 'NONE', *, *, #4274, .F. ) ;
#16596=CARTESIAN_POINT ( 'NONE',  ( 50.00000000000000000, -15.00000000000001954, 10.00000000000008882 ) ) ;
#16606=DIRECTION ( 'NONE',  ( -3.697785493223484080E-32, -0.3420201433256691015, -0.9396926207859082059 ) ) ;
#16607=LINE ( 'NONE', #20055, #11786 ) ;
#16608=CARTESIAN_POINT ( 'NONE',  ( 22.11331769071655984, -8.974600000000002353, 5.000000000000079936 ) ) ;
#16609=ORIENTED_EDGE ( 'NONE', *, *, #1544, .T. ) ;
#16616=ORIENTED_EDGE ( 'NONE', *, *, #13888, .F. ) ;
#16620=VECTOR ( 'NONE', #20771, 1000.000000000000000 ) ;
#16623=ORIENTED_EDGE ( 'NONE', *, *, #9134, .T. ) ;
#16625=DIRECTION ( 'NONE',  ( 0.000000000000000000, 0.000000000000000000, 1.000000000000000000 ) ) ;
#16627=DIRECTION ( 'NONE',  ( -1.000000000000000000, -7.703719777548943412E-32, 0.000000000000000000 ) ) ;
#16644=ORIENTED_EDGE ( 'NONE', *, *, #9816, .T. ) ;
#16646=LINE ( 'NONE', #224, #297 ) ;
#16652=EDGE_CURVE ( 'NONE', #13240, #4980, #10387, .T. ) ;
#16653=ORIENTED_EDGE ( 'NONE', *, *, #17584, .F. ) ;
#16654=AXIS2_PLACEMENT_3D ( 'NONE', #497, #16920, #2160 ) ;
#16666=VECTOR ( 'NONE', #15100, 1000.000000000000000 ) ;
#16673=DIRECTION ( 'NONE',  ( -0.3420201433256622181, 0.9396926207859106484, 1.232595164407828100E-31 ) ) ;
#16700=FACE_OUTER_BOUND ( 'NONE', #6186, .T. ) ;
#16701=ORIENTED_EDGE ( 'NONE', *, *, #22400, .T. ) ;
#16704=EDGE_CURVE ( 'NONE', #3848, #17653, #10030, .T. ) ;
#16706=ORIENTED_EDGE ( 'NONE', *, *, #20670, .F. ) ;
#16712=CARTESIAN_POINT ( 'NONE',  ( 45.00000000000000000, -2.399706452296378245, 55.00000000000021316 ) ) ;
#16719=VECTOR ( 'NONE', #17859, 1000.000000000000000 ) ;
#16741=EDGE_LOOP ( 'NONE', ( #18756, #3602, #21771, #4886 ) ) ;
#16743=AXIS2_PLACEMENT_3D ( 'NONE', #10790, #16163, #5017 ) ;
#16746=CARTESIAN_POINT ( 'NONE',  ( -19.99999999999999645, -9.000000000000003553, 10.00000000000008882 ) ) ;
#16761=CARTESIAN_POINT ( 'NONE',  ( 22.71892870323381075, -9.000000000000005329, 5.000000000000079936 ) ) ;
#16763=VERTEX_POINT ( 'NONE', #4614 ) ;
#16772=DIRECTION ( 'NONE',  ( -0.000000000000000000, 0.000000000000000000, -1.000000000000000000 ) ) ;
#16774=DIRECTION ( 'NONE',  ( 0.3420201433256622181, 0.9396926207859107594, -6.162975822039141593E-32 ) ) ;
#16782=EDGE_CURVE ( 'NONE', #2702, #14967, #2556, .T. ) ;
#16794=PRODUCT_CONTEXT ( 'NONE', #17102, 'mechanical' ) ;
#16796=VERTEX_POINT ( 'NONE', #11948 ) ;
#16803=VECTOR ( 'NONE', #21762, 1000.000000000000000 ) ;
#16810=DIRECTION ( 'NONE',  ( 0.3420201433256622181, 0.9396926207859107594, -6.162975822039141593E-32 ) ) ;
#16818=VECTOR ( 'NONE', #8156, 1000.000000000000000 ) ;
#16819=CARTESIAN_POINT ( 'NONE',  ( 50.00000000000000000, 18.33638201715224270, 11.21434374438452508 ) ) ;
#16822=DIRECTION ( 'NONE',  ( 0.000000000000000000, 0.000000000000000000, -1.000000000000000000 ) ) ;
#16842=VECTOR ( 'NONE', #2060, 1000.000000000000000 ) ;
#16847=DIRECTION ( 'NONE',  ( -0.9396926207859107594, -0.3420201433256623291, 1.540743955509804830E-32 ) ) ;
#16863=ORIENTED_EDGE ( 'NONE', *, *, #22860, .T. ) ;
#16869=DIRECTION ( 'NONE',  ( 0.9396926207859107594, -0.3420201433256623291, 3.697785493223492838E-32 ) ) ;
#16875=DIRECTION ( 'NONE',  ( 0.000000000000000000, 0.000000000000000000, 1.000000000000000000 ) ) ;
#16877=DIRECTION ( 'NONE',  ( 0.3420201433256622736, -0.9396926207859106484, -1.232595164407828100E-31 ) ) ;
#16878=CARTESIAN_POINT ( 'NONE',  ( -19.99999999999999645, -9.000000000000003553, 10.00000000000008882 ) ) ;
#16880=ORIENTED_EDGE ( 'NONE', *, *, #5850, .T. ) ;
#16885=ADVANCED_FACE ( 'NONE', ( #5637 ), #9260, .T. ) ;
#16889=DIRECTION ( 'NONE',  ( 0.000000000000000000, 0.000000000000000000, 1.000000000000000000 ) ) ;
#16890=PLANE ( 'NONE',  #1041 ) ;
#16899=FACE_OUTER_BOUND ( 'NONE', #10665, .T. ) ;
#16906=CARTESIAN_POINT ( 'NONE',  ( 1.546713180332750293, -11.25000000000000355, 5.000000000000079936 ) ) ;
#16913=ORIENTED_EDGE ( 'NONE', *, *, #19484, .F. ) ;
#16920=DIRECTION ( 'NONE',  ( 7.087422195345011518E-32, 1.000000000000000000, -0.000000000000000000 ) ) ;
#16930=PLANE ( 'NONE',  #8438 ) ;
#16932=CARTESIAN_POINT ( 'NONE',  ( 1.546713180332750293, -11.25000000000000355, 5.000000000000079936 ) ) ;
#16937=ORIENTED_EDGE ( 'NONE', *, *, #5419, .T. ) ;
#16949=ADVANCED_FACE ( 'NONE', ( #1679 ), #3955, .T. ) ;
#16952=CARTESIAN_POINT ( 'NONE',  ( 30.70991776966726405, -11.25000000000000355, 5.000000000000079936 ) ) ;
#16962=DIRECTION ( 'NONE',  ( 0.3420201433256622181, -0.9396926207859107594, 0.000000000000000000 ) ) ;
#16967=VERTEX_POINT ( 'NONE', #14768 ) ;
#16973=CARTESIAN_POINT ( 'NONE',  ( 44.09522139676619901, -9.000000000000003553, 10.00454388062671640 ) ) ;
#16979=LINE ( 'NONE', #18411, #9987 ) ;
#16983=PRODUCT ( 'Gripper Jaw with Integrated Rack', 'Gripper Jaw with Integrated Rack', '', ( #16794 ) ) ;
#16995=ORIENTED_EDGE ( 'NONE', *, *, #19514, .T. ) ;
#16997=CARTESIAN_POINT ( 'NONE',  ( 46.41788101966725577, -11.25000000000000355, 5.000000000000079936 ) ) ;
#16998=VERTEX_POINT ( 'NONE', #483 ) ;
#17002=DIRECTION ( 'NONE',  ( 0.000000000000000000, 0.000000000000000000, 1.000000000000000000 ) ) ;
#17007=ADVANCED_FACE ( 'NONE', ( #18919 ), #6117, .F. ) ;
#17010=CARTESIAN_POINT ( 'NONE',  ( 25.25491034071656316, -8.974600000000002353, 10.00000000000008882 ) ) ;
#17011=DIRECTION ( 'NONE',  ( 0.3420201433256622736, 0.9396926207859106484, 0.000000000000000000 ) ) ;
#17019=CARTESIAN_POINT ( 'NONE',  ( 50.00000000000000000, 15.00000000000001954, 10.00000000000008882 ) ) ;
#17024=VECTOR ( 'NONE', #2745, 1000.000000000000000 ) ;
#17025=LINE ( 'NONE', #599, #6638 ) ;
#17029=ORIENTED_EDGE ( 'NONE', *, *, #6733, .T. ) ;
#17040=VECTOR ( 'NONE', #18664, 1000.000000000000114 ) ;
#17042=VECTOR ( 'NONE', #19826, 1000.000000000000114 ) ;
#17050=LINE ( 'NONE', #4341, #19660 ) ;
#17080=EDGE_CURVE ( 'NONE', #1856, #23288, #20935, .T. ) ;
#17081=LINE ( 'NONE', #654, #16620 ) ;
#17089=EDGE_CURVE ( 'NONE', #5711, #10249, #10085, .T. ) ;
#17092=CARTESIAN_POINT ( 'NONE',  ( 44.00000000000000711, -9.261618637464055226, 10.00000000000008882 ) ) ;
#17095=ORIENTED_EDGE ( 'NONE', *, *, #14379, .T. ) ;
#17099=DIRECTION ( 'NONE',  ( -1.000000000000000000, -7.703719777548943412E-32, 0.000000000000000000 ) ) ;
#17101=DIRECTION ( 'NONE',  ( 1.000000000000000000, 7.703719777548943412E-32, 0.000000000000000000 ) ) ;
#17102=APPLICATION_CONTEXT ( 'automotive_design' ) ;
#17106=CARTESIAN_POINT ( 'NONE',  ( 3.860127959283449428, -8.974600000000002353, 5.000000000000079936 ) ) ;
#17107=VERTEX_POINT ( 'NONE', #11539 ) ;
#17109=CARTESIAN_POINT ( 'NONE',  ( 3.263761790716562139, -8.974600000000002353, 5.000000000000079936 ) ) ;
#17110=CARTESIAN_POINT ( 'NONE',  ( -19.99999999999999645, -9.000000000000003553, 5.000000000000079936 ) ) ;
#17112=VECTOR ( 'NONE', #11218, 1000.000000000000000 ) ;
#17115=CARTESIAN_POINT ( 'NONE',  ( 31.53809564071656624, -8.974600000000002353, 5.000000000000079936 ) ) ;
#17118=LINE ( 'NONE', #925, #14462 ) ;
#17119=ORIENTED_EDGE ( 'NONE', *, *, #15388, .T. ) ;
#17151=ADVANCED_FACE ( 'NONE', ( #7696 ), #20469, .F. ) ;
#17152=ORIENTED_EDGE ( 'NONE', *, *, #21526, .T. ) ;
#17156=EDGE_CURVE ( 'NONE', #3825, #14828, #2276, .T. ) ;
#17162=VECTOR ( 'NONE', #18210, 1000.000000000000000 ) ;
#17164=FACE_OUTER_BOUND ( 'NONE', #9981, .T. ) ;
#17167=AXIS2_PLACEMENT_3D ( 'NONE', #340, #7676, #464 ) ;
#17172=DIRECTION ( 'NONE',  ( -1.000000000000000000, -7.703719777548943412E-32, 0.000000000000000000 ) ) ;
#17174=LINE ( 'NONE', #22419, #7845 ) ;
#17191=VECTOR ( 'NONE', #16008, 1000.000000000000000 ) ;
#17203=LINE ( 'NONE', #5817, #2486 ) ;
#17206=DIRECTION ( 'NONE',  ( -1.000000000000000000, -7.703719777548943412E-32, 0.000000000000000000 ) ) ;
#17207=ORIENTED_EDGE ( 'NONE', *, *, #9262, .F. ) ;
#17214=ORIENTED_EDGE ( 'NONE', *, *, #15350, .F. ) ;
#17228=DIRECTION ( 'NONE',  ( 6.779273404243053781E-32, 0.9396926207859083169, -0.3420201433256691015 ) ) ;
#17236=CARTESIAN_POINT ( 'NONE',  ( 50.00000000000000711, -15.00000000000001954, 5.000000000000079936 ) ) ;
#17254=LINE ( 'NONE', #15467, #1051 ) ;
#17264=FACE_OUTER_BOUND ( 'NONE', #3604, .T. ) ;
#17272=ORIENTED_EDGE ( 'NONE', *, *, #2644, .F. ) ;
#17275=LINE ( 'NONE', #4569, #17435 ) ;
#17288=EDGE_CURVE ( 'NONE', #15383, #4326, #3337, .T. ) ;
#17290=CARTESIAN_POINT ( 'NONE',  ( 45.00000000000000000, 10.00000000000001599, 34.11836509645781490 ) ) ;
#17296=VERTEX_POINT ( 'NONE', #15595 ) ;
#17304=CARTESIAN_POINT ( 'NONE',  ( 2.435583919667260400, -11.25000000000000355, 5.000000000000079936 ) ) ;
#17317=EDGE_CURVE ( 'NONE', #13840, #13272, #12239, .T. ) ;
#17325=LINE ( 'NONE', #22240, #18479 ) ;
#17335=VERTEX_POINT ( 'NONE', #13909 ) ;
#17337=AXIS2_PLACEMENT_3D ( 'NONE', #9263, #20238, #3845 ) ;
#17341=EDGE_CURVE ( 'NONE', #14967, #23165, #21408, .T. ) ;
#17342=EDGE_LOOP ( 'NONE', ( #16623, #15492, #7544, #15289 ) ) ;
#17343=DIRECTION ( 'NONE',  ( 5.546678239835225025E-32, 0.3420201433256690460, 0.9396926207859082059 ) ) ;
#17360=EDGE_LOOP ( 'NONE', ( #12865, #15824 ) ) ;
#17366=DIRECTION ( 'NONE',  ( 1.000000000000000000, 7.703719777548943412E-32, 0.000000000000000000 ) ) ;
#17380=LINE ( 'NONE', #951, #2690 ) ;
#17388=VERTEX_POINT ( 'NONE', #10562 ) ;
#17394=EDGE_CURVE ( 'NONE', #15383, #17500, #19858, .T. ) ;
#17399=VECTOR ( 'NONE', #17652, 1000.000000000000000 ) ;
#17408=LINE ( 'NONE', #8306, #20255 ) ;
#17411=PLANE ( 'NONE',  #22341 ) ;
#17435=VECTOR ( 'NONE', #8291, 1000.000000000000114 ) ;
#17455=DIRECTION ( 'NONE',  ( 0.3420201433256622181, 0.9396926207859107594, -6.162975822039141593E-32 ) ) ;
#17458=EDGE_CURVE ( 'NONE', #2919, #12703, #9231, .T. ) ;
#17464=PLANE ( 'NONE',  #9570 ) ;
#17467=LINE ( 'NONE', #13764, #3994 ) ;
#17472=CARTESIAN_POINT ( 'NONE',  ( -19.99999999999999645, -9.000000000000003553, 5.000000000000079936 ) ) ;
#17496=ORIENTED_EDGE ( 'NONE', *, *, #7139, .F. ) ;
#17498=CARTESIAN_POINT ( 'NONE',  ( 23.53786173033275375, -11.25000000000000355, 10.00000000000008882 ) ) ;
#17500=VERTEX_POINT ( 'NONE', #11738 ) ;
#17528=ORIENTED_EDGE ( 'NONE', *, *, #3933, .F. ) ;
#17531=ORIENTED_EDGE ( 'NONE', *, *, #12425, .F. ) ;
#17542=CARTESIAN_POINT ( 'NONE',  ( -4.736472119667250347, -11.25000000000000355, 10.00000000000008882 ) ) ;
#17543=AXIS2_PLACEMENT_3D ( 'NONE', #23260, #10488, #2789 ) ;
#17544=EDGE_CURVE ( 'NONE', #21867, #4634, #563, .T. ) ;
#17562=ORIENTED_EDGE ( 'NONE', *, *, #16652, .F. ) ;
#17567=ORIENTED_EDGE ( 'NONE', *, *, #2796, .F. ) ;
#17570=CARTESIAN_POINT ( 'NONE',  ( 118.3095189484530181, 10.00000000000001599, 15.00000000000003020 ) ) ;
#17578=PRODUCT_DEFINITION_FORMATION_WITH_SPECIFIED_SOURCE ( 'ANY', '', #16983, .NOT_KNOWN. ) ;
#17584=EDGE_CURVE ( 'NONE', #22779, #17107, #4286, .T. ) ;
#17588=LINE ( 'NONE', #22605, #12868 ) ;
#17616=VECTOR ( 'NONE', #19132, 1000.000000000000000 ) ;
#17626=LINE ( 'NONE', #10333, #22185 ) ;
#17632=CARTESIAN_POINT ( 'NONE',  ( -19.99999999999999645, -9.000000000000003553, 5.000000000000079936 ) ) ;
#17642=EDGE_CURVE ( 'NONE', #10312, #476, #13986, .T. ) ;
#17647=CARTESIAN_POINT ( 'NONE',  ( 50.00000000000000000, 10.00000000000001599, 17.50000000000003197 ) ) ;
#17651=EDGE_LOOP ( 'NONE', ( #15732, #23056, #17766, #7708 ) ) ;
#17652=DIRECTION ( 'NONE',  ( 1.000000000000000000, 7.703719777548943412E-32, 0.000000000000000000 ) ) ;
#17653=VERTEX_POINT ( 'NONE', #2590 ) ;
#17657=ORIENTED_EDGE ( 'NONE', *, *, #4796, .F. ) ;
#17661=ORIENTED_EDGE ( 'NONE', *, *, #4095, .T. ) ;
#17665=DIRECTION ( 'NONE',  ( 1.000000000000000000, 7.703719777548943412E-32, 0.000000000000000000 ) ) ;
#17681=ORIENTED_EDGE ( 'NONE', *, *, #19737, .F. ) ;
#17682=ADVANCED_FACE ( 'NONE', ( #14985 ), #22604, .F. ) ;
#17701=ORIENTED_EDGE ( 'NONE', *, *, #19807, .F. ) ;
#17707=DIRECTION ( 'NONE',  ( 0.000000000000000000, 0.000000000000000000, 1.000000000000000000 ) ) ;
#17708=DIRECTION ( 'NONE',  ( 0.3420201433256622181, 0.9396926207859107594, -6.162975822039141593E-32 ) ) ;
#17711=ORIENTED_EDGE ( 'NONE', *, *, #21922, .F. ) ;
#17715=EDGE_CURVE ( 'NONE', #7167, #7410, #1378, .T. ) ;
#17729=CARTESIAN_POINT ( 'NONE',  ( 44.09522139676619901, -9.000000000000007105, 5.000000000000079936 ) ) ;
#17737=ORIENTED_EDGE ( 'NONE', *, *, #12027, .T. ) ;
#17740=CARTESIAN_POINT ( 'NONE',  ( -19.99999999999999645, -15.00000000000001954, 10.00000000000008882 ) ) ;
#17744=DIRECTION ( 'NONE',  ( 0.000000000000000000, 0.000000000000000000, 1.000000000000000000 ) ) ;
#17746=DIRECTION ( 'NONE',  ( -7.087422195345011518E-32, -1.000000000000000000, 0.000000000000000000 ) ) ;
#17750=CARTESIAN_POINT ( 'NONE',  ( 50.00000000000000000, -10.00000000000001954, 12.50000000000002665 ) ) ;
#17756=LINE ( 'NONE', #6741, #2300 ) ;
#17757=ORIENTED_EDGE ( 'NONE', *, *, #17715, .T. ) ;
#17765=LINE ( 'NONE', #4597, #1823 ) ;
#17766=ORIENTED_EDGE ( 'NONE', *, *, #13112, .F. ) ;
#17771=AXIS2_PLACEMENT_3D ( 'NONE', #3523, #16231, #6770 ) ;
#17792=FACE_OUTER_BOUND ( 'NONE', #4029, .T. ) ;
#17803=VECTOR ( 'NONE', #7156, 1000.000000000000000 ) ;
#17813=CARTESIAN_POINT ( 'NONE',  ( -6.989194030332740226, -11.25000000000000355, 10.00000000000008882 ) ) ;
#17830=EDGE_LOOP ( 'NONE', ( #16055, #23563, #22671, #1131, #21290, #11995, #15075, #7324, #8953, #13742, #7487, #5179, #3229, #10922, #17701, #5096, #4440, #8601, #11803, #10368, #23472, #307, #2092, #22814, #22035, #14390, #23248, #13515, #7905, #5794, #5090, #21940, #6595, #19464, #6985, #22369, #14601, #23026, #13196, #7910, #5468, #6351, #21708, #21243, #5060, #11392, #14394, #72, #15469, #4741, #15399, #4675, #10096, #20085, #6718, #18006, #10974, #3439, #22953, #21863, #5236, #22464, #2284, #18659, #17029, #14644, #10579, #3142, #12700, #14396, #8692, #12178, #10776, #5119, #3879, #15838, #11300, #23375, #13490, #1106, #1195, #5472, #11514, #9628, #10892 ) ) ;
#17833=ADVANCED_FACE ( 'NONE', ( #16023 ), #20904, .F. ) ;
#17843=DIRECTION ( 'NONE',  ( 1.000000000000000000, 0.000000000000000000, 0.000000000000000000 ) ) ;
#17845=VERTEX_POINT ( 'NONE', #3186 ) ;
#17853=VERTEX_POINT ( 'NONE', #11974 ) ;
#17859=DIRECTION ( 'NONE',  ( 0.000000000000000000, 0.000000000000000000, 1.000000000000000000 ) ) ;
#17861=EDGE_CURVE ( 'NONE', #21099, #18371, #19354, .T. ) ;
#17873=VECTOR ( 'NONE', #10615, 1000.000000000000114 ) ;
#17874=CARTESIAN_POINT ( 'NONE',  ( -16.41397198033274307, -11.25000000000000355, 10.00000000000008882 ) ) ;
#17880=FACE_OUTER_BOUND ( 'NONE', #17651, .T. ) ;
#17887=AXIS2_PLACEMENT_3D ( 'NONE', #15814, #825, #15705 ) ;
#17893=VECTOR ( 'NONE', #20451, 1000.000000000000114 ) ;
#17907=CARTESIAN_POINT ( 'NONE',  ( -8.706242640716551406, -8.974600000000002353, 5.000000000000079936 ) ) ;
#17912=VERTEX_POINT ( 'NONE', #3308 ) ;
#17917=LINE ( 'NONE', #8707, #9104 ) ;
#17920=AXIS2_PLACEMENT_3D ( 'NONE', #13077, #20334, #11273 ) ;
#17924=CYLINDRICAL_SURFACE ( 'NONE', #4566, 5.000000000000011546 ) ;
#17930=VECTOR ( 'NONE', #437, 1000.000000000000000 ) ;
#17934=CARTESIAN_POINT ( 'NONE',  ( 45.00000000000000000, 14.69846310392956745, 35.82846581308617573 ) ) ;
#17941=EDGE_CURVE ( 'NONE', #5492, #21989, #12798, .T. ) ;
#17946=VECTOR ( 'NONE', #18268, 1000.000000000000114 ) ;
#17947=CARTESIAN_POINT ( 'NONE',  ( 50.00000000000000000, 15.00000000000003375, 34.11836509645780069 ) ) ;
#17949=ORIENTED_EDGE ( 'NONE', *, *, #20871, .F. ) ;
#17950=CARTESIAN_POINT ( 'NONE',  ( -6.989194030332740226, -11.25000000000000355, 10.00000000000008882 ) ) ;
#17955=DIRECTION ( 'NONE',  ( 0.3420201433256622181, 0.9396926207859107594, -6.162975822039141593E-32 ) ) ;
#17963=DIRECTION ( 'NONE',  ( 7.087422195345011518E-32, 1.000000000000000000, -0.000000000000000000 ) ) ;
#17966=VECTOR ( 'NONE', #18130, 1000.000000000000000 ) ;
#17972=( BOUNDED_CURVE ( )  B_SPLINE_CURVE ( 3, ( #9540, #7145, #10980, #7270 ),
 .UNSPECIFIED., .F., .F. ) 
 B_SPLINE_CURVE_WITH_KNOTS ( ( 4, 4 ),
 ( 5.501996899079006020, 6.283185307179586232 ),
 .UNSPECIFIED. ) 
 CURVE ( )  GEOMETRIC_REPRESENTATION_ITEM ( )  RATIONAL_B_SPLINE_CURVE ( ( 1.000000000000000000, 0.9497886580611611951, 0.9497886580611611951, 1.000000000000000000 ) ) 
 REPRESENTATION_ITEM ( '' )  );
#17973=EDGE_CURVE ( 'NONE', #5711, #14744, #21497, .T. ) ;
#17988=CARTESIAN_POINT ( 'NONE',  ( 0.7185353092834488864, -8.974600000000002353, 5.000000000000079936 ) ) ;
#17994=ORIENTED_EDGE ( 'NONE', *, *, #12316, .T. ) ;
#17999=VERTEX_POINT ( 'NONE', #19704 ) ;
#18003=EDGE_CURVE ( 'NONE', #12149, #23165, #16259, .T. ) ;
#18006=ORIENTED_EDGE ( 'NONE', *, *, #16451, .F. ) ;
#18009=EDGE_CURVE ( 'NONE', #10792, #11370, #21736, .T. ) ;
#18021=ORIENTED_EDGE ( 'NONE', *, *, #22231, .F. ) ;
#18023=PLANE ( 'NONE',  #17771 ) ;
#18028=CARTESIAN_POINT ( 'NONE',  ( 45.00000000000000000, -2.399706452296378245, 55.00000000000021316 ) ) ;
#18035=CARTESIAN_POINT ( 'NONE',  ( 32.14370665323380649, -9.000000000000001776, 10.00000000000008882 ) ) ;
#18039=DIRECTION ( 'NONE',  ( 0.3420201433256622736, -0.9396926207859106484, -1.232595164407828100E-31 ) ) ;
#18046=DIRECTION ( 'NONE',  ( 0.000000000000000000, 0.000000000000000000, 1.000000000000000000 ) ) ;
#18051=DIRECTION ( 'NONE',  ( -0.3420201433256622181, 0.9396926207859106484, 1.232595164407828100E-31 ) ) ;
#18053=CARTESIAN_POINT ( 'NONE',  ( 118.3095189484530181, 2.399706452296379577, 55.00000000000021316 ) ) ;
#18054=VERTEX_POINT ( 'NONE', #4373 ) ;
#18058=ORIENTED_EDGE ( 'NONE', *, *, #11500, .F. ) ;
#18069=LINE ( 'NONE', #1649, #9177 ) ;
#18078=CARTESIAN_POINT ( 'NONE',  ( -3.028668353233797905, -9.000000000000003553, 5.000000000000079936 ) ) ;
#18091=CARTESIAN_POINT ( 'NONE',  ( 40.13469571966727045, -11.25000000000000355, 10.00000000000008882 ) ) ;
#18093=VECTOR ( 'NONE', #13380, 1000.000000000000114 ) ;
#18104=CARTESIAN_POINT ( 'NONE',  ( 25.24566549676620397, -9.000000000000001776, 10.00000000000008882 ) ) ;
#18105=EDGE_LOOP ( 'NONE', ( #9818, #17496, #11005, #12045 ) ) ;
#18112=EDGE_CURVE ( 'NONE', #3848, #21099, #17203, .T. ) ;
#18115=VECTOR ( 'NONE', #18978, 1000.000000000000000 ) ;
#18130=DIRECTION ( 'NONE',  ( 0.000000000000000000, 0.000000000000000000, -1.000000000000000000 ) ) ;
#18149=EDGE_CURVE ( 'NONE', #13840, #8586, #564, .T. ) ;
#18154=ADVANCED_FACE ( 'NONE', ( #5968 ), #16318, .T. ) ;
#18157=( NAMED_UNIT ( * ) SI_UNIT ( $, .STERADIAN. ) SOLID_ANGLE_UNIT ( ) );
#18160=DIRECTION ( 'NONE',  ( 0.3420201433256622736, -0.9396926207859106484, -1.232595164407828100E-31 ) ) ;
#18161=ORIENTED_EDGE ( 'NONE', *, *, #943, .F. ) ;
#18163=DIRECTION ( 'NONE',  ( 1.000000000000000000, 7.703719777548943412E-32, 0.000000000000000000 ) ) ;
#18164=PLANE ( 'NONE',  #6690 ) ;
#18175=SHAPE_REPRESENTATION ( 'Gripper Jaw with Integrated Rack', ( #7318 ), #28 ) ;
#18178=CARTESIAN_POINT ( 'NONE',  ( 15.83013239071656741, -8.974600000000002353, 5.000000000000079936 ) ) ;
#18180=CARTESIAN_POINT ( 'NONE',  ( 50.38765154071656838, -8.974600000000002353, 5.000000000000079936 ) ) ;
#18181=ORIENTED_EDGE ( 'NONE', *, *, #12604, .F. ) ;
#18184=PLANE ( 'NONE',  #739 ) ;
#18186=CARTESIAN_POINT ( 'NONE',  ( -16.41397198033274307, -11.25000000000000355, 10.00000000000008882 ) ) ;
#18187=CARTESIAN_POINT ( 'NONE',  ( 49.55947366966726264, -11.25000000000000355, 5.000000000000079936 ) ) ;
#18195=EDGE_CURVE ( 'NONE', #16998, #21720, #9586, .T. ) ;
#18196=ADVANCED_FACE ( 'NONE', ( #19241 ), #19130, .F. ) ;
#18197=ORIENTED_EDGE ( 'NONE', *, *, #20638, .F. ) ;
#18204=VECTOR ( 'NONE', #18163, 1000.000000000000000 ) ;
#18210=DIRECTION ( 'NONE',  ( -1.000000000000000000, -7.703719777548943412E-32, 0.000000000000000000 ) ) ;
#18219=CARTESIAN_POINT ( 'NONE',  ( -12.45344630323380208, -9.000000000000003553, 5.000000000000079936 ) ) ;
#18233=VECTOR ( 'NONE', #16822, 1000.000000000000000 ) ;
#18241=AXIS2_PLACEMENT_3D ( 'NONE', #9084, #13036, #3778 ) ;
#18244=LINE ( 'NONE', #10968, #15498 ) ;
#18245=ORIENTED_EDGE ( 'NONE', *, *, #6725, .T. ) ;
#18250=VERTEX_POINT ( 'NONE', #10058 ) ;
#18254=VERTEX_POINT ( 'NONE', #8013 ) ;
#18265=CARTESIAN_POINT ( 'NONE',  ( -5.555405146766190683, -9.000000000000005329, 5.000000000000079936 ) ) ;
#18268=DIRECTION ( 'NONE',  ( -0.3420201433256622181, 0.9396926207859106484, 1.232595164407828100E-31 ) ) ;
#18282=ADVANCED_FACE ( 'NONE', ( #19355 ), #2594, .F. ) ;
#18294=LINE ( 'NONE', #1878, #22080 ) ;
#18301=DIRECTION ( 'NONE',  ( 0.000000000000000000, 0.000000000000000000, -1.000000000000000000 ) ) ;
#18305=LINE ( 'NONE', #1887, #11285 ) ;
#18307=DIRECTION ( 'NONE',  ( -2.465190328815656418E-32, -0.3420201433256690460, 0.9396926207859083169 ) ) ;
#18317=FACE_OUTER_BOUND ( 'NONE', #1692, .T. ) ;
#18323=EDGE_CURVE ( 'NONE', #6488, #2752, #17588, .T. ) ;
#18331=ADVANCED_FACE ( 'NONE', ( #6447 ), #8372, .F. ) ;
#18349=SHAPE_DEFINITION_REPRESENTATION ( #7618, #18175 ) ;
#18353=ORIENTED_EDGE ( 'NONE', *, *, #23667, .F. ) ;
#18357=MECHANICAL_DESIGN_GEOMETRIC_PRESENTATION_REPRESENTATION('',(#6504),#1129);
#18364=AXIS2_PLACEMENT_3D ( 'NONE', #8187, #15500, #20847 ) ;
#18371=VERTEX_POINT ( 'NONE', #20795 ) ;
#18378=CARTESIAN_POINT ( 'NONE',  ( 45.00000000000000000, 15.00000000000001954, 10.00000000000008882 ) ) ;
#18384=CIRCLE ( 'NONE', #21817, 2.500000000000007550 ) ;
#18394=DIRECTION ( 'NONE',  ( 1.000000000000000000, 7.703719777548943412E-32, 0.000000000000000000 ) ) ;
#18398=FACE_OUTER_BOUND ( 'NONE', #1240, .T. ) ;
#18402=LINE ( 'NONE', #9562, #2578 ) ;
#18406=EDGE_LOOP ( 'NONE', ( #16937, #432, #705, #15552 ) ) ;
#18411=CARTESIAN_POINT ( 'NONE',  ( 10.97149113033275114, -11.25000000000000355, 5.000000000000079936 ) ) ;
#18422=VERTEX_POINT ( 'NONE', #23432 ) ;
#18432=LINE ( 'NONE', #5745, #11405 ) ;
#18435=VERTEX_POINT ( 'NONE', #5349 ) ;
#18436=ADVANCED_FACE ( 'NONE', ( #20052 ), #21737, .F. ) ;
#18457=ORIENTED_EDGE ( 'NONE', *, *, #18863, .F. ) ;
#18459=ORIENTED_EDGE ( 'NONE', *, *, #12655, .T. ) ;
#18473=CARTESIAN_POINT ( 'NONE',  ( -6.170261003233799890, -9.000000000000005329, 5.000000000000079936 ) ) ;
#18479=VECTOR ( 'NONE', #890, 1000.000000000000000 ) ;
#18482=VERTEX_POINT ( 'NONE', #5000 ) ;
#18493=EDGE_LOOP ( 'NONE', ( #21315, #8839, #8758, #20178 ) ) ;
#18494=CARTESIAN_POINT ( 'NONE',  ( -7.878064769667250999, -11.25000000000000355, 10.00000000000008882 ) ) ;
#18497=LINE ( 'NONE', #22072, #4345 ) ;
#18506=DIRECTION ( 'NONE',  ( 0.000000000000000000, 5.754033390038007439E-16, 1.000000000000000000 ) ) ;
#18507=CARTESIAN_POINT ( 'NONE',  ( 35.28529930323381336, -9.000000000000003553, 5.000000000000079936 ) ) ;
#18509=VERTEX_POINT ( 'NONE', #23551 ) ;
#18516=ORIENTED_EDGE ( 'NONE', *, *, #20734, .F. ) ;
#18521=VECTOR ( 'NONE', #21318, 1000.000000000000000 ) ;
#18524=ORIENTED_EDGE ( 'NONE', *, *, #11998, .T. ) ;
#18533=VERTEX_POINT ( 'NONE', #23183 ) ;
#18538=ORIENTED_EDGE ( 'NONE', *, *, #21526, .F. ) ;
#18539=CARTESIAN_POINT ( 'NONE',  ( 28.99286915928345110, -8.974600000000002353, 5.000000000000079936 ) ) ;
#18540=LINE ( 'NONE', #22006, #9863 ) ;
#18545=ORIENTED_EDGE ( 'NONE', *, *, #19878, .F. ) ;
#18546=LINE ( 'NONE', #345, #21358 ) ;
#18561=EDGE_CURVE ( 'NONE', #18607, #4290, #7514, .T. ) ;
#18571=VECTOR ( 'NONE', #22837, 1000.000000000000000 ) ;
#18578=EDGE_LOOP ( 'NONE', ( #19928, #13863, #2292, #3374 ) ) ;
#18580=ORIENTED_EDGE ( 'NONE', *, *, #452, .F. ) ;
#18587=EDGE_CURVE ( 'NONE', #2784, #6494, #6058, .T. ) ;
#18593=EDGE_CURVE ( 'NONE', #19389, #13563, #67, .T. ) ;
#18595=EDGE_CURVE ( 'NONE', #12636, #7229, #5700, .T. ) ;
#18599=DIRECTION ( 'NONE',  ( -1.000000000000000000, -7.703719777548943412E-32, 0.000000000000000000 ) ) ;
#18607=VERTEX_POINT ( 'NONE', #22207 ) ;
#18609=DIRECTION ( 'NONE',  ( 1.000000000000000000, 7.703719777548943412E-32, 0.000000000000000000 ) ) ;
#18611=EDGE_LOOP ( 'NONE', ( #14333, #15460, #8582, #6098 ) ) ;
#18617=DIRECTION ( 'NONE',  ( -1.000000000000000000, -7.703719777548943412E-32, 0.000000000000000000 ) ) ;
#18619=EDGE_CURVE ( 'NONE', #2759, #7447, #5580, .T. ) ;
#18635=VECTOR ( 'NONE', #1463, 1000.000000000000114 ) ;
#18640=EDGE_LOOP ( 'NONE', ( #15733, #926, #11249, #20802 ) ) ;
#18655=VECTOR ( 'NONE', #19932, 1000.000000000000000 ) ;
#18658=CARTESIAN_POINT ( 'NONE',  ( 45.00000000000000000, 10.00000000000001599, 12.50000000000002842 ) ) ;
#18659=ORIENTED_EDGE ( 'NONE', *, *, #8964, .F. ) ;
#18662=EDGE_LOOP ( 'NONE', ( #10801, #5701, #12755, #17711 ) ) ;
#18664=DIRECTION ( 'NONE',  ( 0.3420201433256622181, 0.9396926207859107594, -6.162975822039141593E-32 ) ) ;
#18676=VECTOR ( 'NONE', #23652, 1000.000000000000000 ) ;
#18678=LINE ( 'NONE', #17010, #4961 ) ;
#18682=ORIENTED_EDGE ( 'NONE', *, *, #2824, .F. ) ;
#18700=VECTOR ( 'NONE', #1389, 1000.000000000000000 ) ;
#18701=ORIENTED_EDGE ( 'NONE', *, *, #2934, .F. ) ;
#18715=FACE_OUTER_BOUND ( 'NONE', #17830, .T. ) ;
#18725=LINE ( 'NONE', #22182, #20811 ) ;
#18743=VECTOR ( 'NONE', #14041, 1000.000000000000000 ) ;
#18745=CARTESIAN_POINT ( 'NONE',  ( 50.00000000000000000, -2.399706452296352932, 60.00000000000021316 ) ) ;
#18756=ORIENTED_EDGE ( 'NONE', *, *, #974, .F. ) ;
#18766=CARTESIAN_POINT ( 'NONE',  ( 0.1221691407165617638, -8.974600000000002353, 5.000000000000079936 ) ) ;
#18786=ORIENTED_EDGE ( 'NONE', *, *, #7628, .F. ) ;
#18789=ORIENTED_EDGE ( 'NONE', *, *, #5765, .F. ) ;
#18796=CARTESIAN_POINT ( 'NONE',  ( 10.97149113033275114, -11.25000000000000355, 10.00000000000008882 ) ) ;
#18800=PLANE ( 'NONE',  #12296 ) ;
#18821=EDGE_LOOP ( 'NONE', ( #5945, #4090, #19976, #13675 ) ) ;
#18822=DIRECTION ( 'NONE',  ( 0.000000000000000000, 0.000000000000000000, 1.000000000000000000 ) ) ;
#18831=CARTESIAN_POINT ( 'NONE',  ( 118.3095189484530181, 15.00000000000001954, 10.00000000000008882 ) ) ;
#18838=LINE ( 'NONE', #13121, #16842 ) ;
#18840=CARTESIAN_POINT ( 'NONE',  ( 24.42673246966726452, -11.25000000000000355, 10.00000000000008882 ) ) ;
#18841=ORIENTED_EDGE ( 'NONE', *, *, #19807, .T. ) ;
#18847=CARTESIAN_POINT ( 'NONE',  ( 50.00000000000000711, -15.00000000000001954, 5.000000000000079936 ) ) ;
#18852=EDGE_CURVE ( 'NONE', #18509, #20280, #17081, .T. ) ;
#18856=DIRECTION ( 'NONE',  ( -1.000000000000000000, -7.703719777548943412E-32, 0.000000000000000000 ) ) ;
#18858=DIRECTION ( 'NONE',  ( 1.000000000000000000, 7.703719777548943412E-32, 0.000000000000000000 ) ) ;
#18863=EDGE_CURVE ( 'NONE', #1035, #21012, #18979, .T. ) ;
#18885=CARTESIAN_POINT ( 'NONE',  ( 24.42673246966726452, -11.25000000000000355, 5.000000000000079936 ) ) ;
#18887=CARTESIAN_POINT ( 'NONE',  ( 118.3095189484530181, -14.69846310392956745, 35.82846581308617573 ) ) ;
#18890=CARTESIAN_POINT ( 'NONE',  ( 32.13446180928345086, -8.974600000000002353, 5.000000000000079936 ) ) ;
#18896=CARTESIAN_POINT ( 'NONE',  ( 33.85151041966726382, -11.25000000000000355, 5.000000000000079936 ) ) ;
#18897=DIRECTION ( 'NONE',  ( 0.000000000000000000, 0.000000000000000000, -1.000000000000000000 ) ) ;
#18900=CARTESIAN_POINT ( 'NONE',  ( 15.82088754676620823, -9.000000000000003553, 5.000000000000079936 ) ) ;
#18903=ORIENTED_EDGE ( 'NONE', *, *, #12326, .T. ) ;
#18919=FACE_OUTER_BOUND ( 'NONE', #11462, .T. ) ;
#18941=AXIS2_PLACEMENT_3D ( 'NONE', #4648, #8698, #23409 ) ;
#18951=LINE ( 'NONE', #23019, #20652 ) ;
#18952=VERTEX_POINT ( 'NONE', #23161 ) ;
#18953=CARTESIAN_POINT ( 'NONE',  ( 12.68853974071656232, -8.974600000000002353, 5.000000000000079936 ) ) ;
#18959=VECTOR ( 'NONE', #18394, 1000.000000000000000 ) ;
#18964=LINE ( 'NONE', #18847, #4124 ) ;
#18966=ORIENTED_EDGE ( 'NONE', *, *, #424, .F. ) ;
#18971=DIRECTION ( 'NONE',  ( 1.000000000000000000, 7.703719777548943412E-32, 0.000000000000000000 ) ) ;
#18978=DIRECTION ( 'NONE',  ( 1.000000000000000000, 7.703719777548943412E-32, 0.000000000000000000 ) ) ;
#18979=LINE ( 'NONE', #9911, #13976 ) ;
#18985=ORIENTED_EDGE ( 'NONE', *, *, #11193, .F. ) ;
#18990=VERTEX_POINT ( 'NONE', #10750 ) ;
#18992=ADVANCED_FACE ( 'NONE', ( #12665 ), #18023, .T. ) ;
#19007=CARTESIAN_POINT ( 'NONE',  ( 5.577176569667260608, -11.25000000000000355, 5.000000000000079936 ) ) ;
#19009=VERTEX_POINT ( 'NONE', #8577 ) ;
#19020=CARTESIAN_POINT ( 'NONE',  ( 31.52885079676620705, -9.000000000000003553, 5.000000000000079936 ) ) ;
#19022=CARTESIAN_POINT ( 'NONE',  ( -8.706242640716551406, -8.974600000000002353, 5.000000000000079936 ) ) ;
#19032=CARTESIAN_POINT ( 'NONE',  ( 12.67929489676620314, -9.000000000000003553, 5.000000000000079936 ) ) ;
#19050=ORIENTED_EDGE ( 'NONE', *, *, #6001, .F. ) ;
#19052=ORIENTED_EDGE ( 'NONE', *, *, #21829, .F. ) ;
#19053=AXIS2_PLACEMENT_3D ( 'NONE', #53, #20279, #20036 ) ;
#19056=ORIENTED_EDGE ( 'NONE', *, *, #13216, .T. ) ;
#19066=PLANE ( 'NONE',  #11244 ) ;
#19074=DIRECTION ( 'NONE',  ( 1.000000000000000000, 7.703719777548943412E-32, 0.000000000000000000 ) ) ;
#19079=VECTOR ( 'NONE', #10443, 1000.000000000000114 ) ;
#19082=LINE ( 'NONE', #17304, #20950 ) ;
#19089=VECTOR ( 'NONE', #11113, 1000.000000000000000 ) ;
#19105=DIRECTION ( 'NONE',  ( -7.087422195345011518E-32, -1.000000000000000000, 0.000000000000000000 ) ) ;
#19110=AXIS2_PLACEMENT_3D ( 'NONE', #22178, #9646, #12881 ) ;
#19117=ORIENTED_EDGE ( 'NONE', *, *, #6725, .F. ) ;
#19118=DIRECTION ( 'NONE',  ( -1.000000000000000000, -7.703719777548943412E-32, 0.000000000000000000 ) ) ;
#19130=PLANE ( 'NONE',  #13632 ) ;
#19132=DIRECTION ( 'NONE',  ( -7.087422195345011518E-32, -1.000000000000000000, 0.000000000000000000 ) ) ;
#19136=AXIS2_PLACEMENT_3D ( 'NONE', #8780, #12853, #12383 ) ;
#19144=ORIENTED_EDGE ( 'NONE', *, *, #21763, .F. ) ;
#19146=LINE ( 'NONE', #699, #3083 ) ;
#19147=CARTESIAN_POINT ( 'NONE',  ( 10.97149113033275114, -11.25000000000000355, 5.000000000000079936 ) ) ;
#19153=DIRECTION ( 'NONE',  ( 0.3420201433256622181, 0.9396926207859107594, -6.162975822039141593E-32 ) ) ;
#19154=EDGE_CURVE ( 'NONE', #14420, #9029, #18725, .T. ) ;
#19175=VECTOR ( 'NONE', #23458, 1000.000000000000000 ) ;
#19176=ORIENTED_EDGE ( 'NONE', *, *, #877, .F. ) ;
#19178=CARTESIAN_POINT ( 'NONE',  ( -7.878064769667250999, -11.25000000000000355, 5.000000000000079936 ) ) ;
#19179=CARTESIAN_POINT ( 'NONE',  ( 37.82128094071656932, -8.974600000000002353, 5.000000000000079936 ) ) ;
#19180=EDGE_CURVE ( 'NONE', #2366, #17335, #18244, .T. ) ;
#19195=ORIENTED_EDGE ( 'NONE', *, *, #903, .T. ) ;
#19213=CARTESIAN_POINT ( 'NONE',  ( 45.00000000000000000, -10.00000000000001599, 34.11836509645782201 ) ) ;
#19218=ADVANCED_FACE ( 'NONE', ( #13589, #15631, #10118, #8089 ), #17411, .F. ) ;
#19224=ORIENTED_EDGE ( 'NONE', *, *, #21666, .T. ) ;
#19226=ORIENTED_EDGE ( 'NONE', *, *, #14664, .T. ) ;
#19227=ORIENTED_EDGE ( 'NONE', *, *, #23437, .F. ) ;
#19230=ORIENTED_EDGE ( 'NONE', *, *, #15865, .T. ) ;
#19238=CARTESIAN_POINT ( 'NONE',  ( 118.3095189484530181, 14.69846310392956745, 35.82846581308617573 ) ) ;
#19241=FACE_OUTER_BOUND ( 'NONE', #5676, .T. ) ;
#19245=PLANE ( 'NONE',  #12361 ) ;
#19256=EDGE_CURVE ( 'NONE', #22731, #375, #17174, .T. ) ;
#19271=CARTESIAN_POINT ( 'NONE',  ( -18.73663160323380339, -9.000000000000003553, 5.000000000000079936 ) ) ;
#19275=FACE_OUTER_BOUND ( 'NONE', #19721, .T. ) ;
#19282=ADVANCED_FACE ( 'NONE', ( #22662 ), #6272, .F. ) ;
#19300=DIRECTION ( 'NONE',  ( 0.9396926207859107594, -0.3420201433256623291, 3.697785493223492838E-32 ) ) ;
#19301=ORIENTED_EDGE ( 'NONE', *, *, #13970, .F. ) ;
#19307=VECTOR ( 'NONE', #13298, 1000.000000000000000 ) ;
#19308=EDGE_CURVE ( 'NONE', #17335, #2869, #15158, .T. ) ;
#19309=ORIENTED_EDGE ( 'NONE', *, *, #3478, .F. ) ;
#19318=DIRECTION ( 'NONE',  ( 0.000000000000000000, 0.000000000000000000, -1.000000000000000000 ) ) ;
#19329=LINE ( 'NONE', #10267, #22559 ) ;
#19331=VERTEX_POINT ( 'NONE', #18840 ) ;
#19334=ORIENTED_EDGE ( 'NONE', *, *, #2197, .F. ) ;
#19339=ORIENTED_EDGE ( 'NONE', *, *, #18595, .F. ) ;
#19340=DIRECTION ( 'NONE',  ( -0.3420201433256622181, 0.9396926207859106484, 1.232595164407828100E-31 ) ) ;
#19341=DIRECTION ( 'NONE',  ( 0.000000000000000000, 0.000000000000000000, 1.000000000000000000 ) ) ;
#19354=LINE ( 'NONE', #1151, #14372 ) ;
#19355=FACE_OUTER_BOUND ( 'NONE', #18611, .T. ) ;
#19360=VERTEX_POINT ( 'NONE', #17874 ) ;
#19369=VECTOR ( 'NONE', #16344, 1000.000000000000000 ) ;
#19374=LINE ( 'NONE', #20931, #19841 ) ;
#19389=VERTEX_POINT ( 'NONE', #6626 ) ;
#19393=VERTEX_POINT ( 'NONE', #23489 ) ;
#19399=DIRECTION ( 'NONE',  ( 0.3420201433256622181, 0.9396926207859107594, -6.162975822039141593E-32 ) ) ;
#19402=CARTESIAN_POINT ( 'NONE',  ( 6.396109596766202721, -9.000000000000003553, 5.000000000000079936 ) ) ;
#19404=LINE ( 'NONE', #3487, #22503 ) ;
#19406=AXIS2_PLACEMENT_3D ( 'NONE', #10078, #17366, #4422 ) ;
#19412=DIRECTION ( 'NONE',  ( 0.3420201433256622181, -0.9396926207859107594, 0.000000000000000000 ) ) ;
#19425=ORIENTED_EDGE ( 'NONE', *, *, #18561, .T. ) ;
#19433=VECTOR ( 'NONE', #8023, 1000.000000000000114 ) ;
#19440=EDGE_CURVE ( 'NONE', #12636, #8828, #23247, .T. ) ;
#19443=EDGE_CURVE ( 'NONE', #375, #20062, #21441, .T. ) ;
#19446=VECTOR ( 'NONE', #6732, 1000.000000000000000 ) ;
#19450=VERTEX_POINT ( 'NONE', #15751 ) ;
#19454=CARTESIAN_POINT ( 'NONE',  ( 9.537702246766199821, -9.000000000000005329, 10.00000000000008882 ) ) ;
#19464=ORIENTED_EDGE ( 'NONE', *, *, #4733, .T. ) ;
#19469=VECTOR ( 'NONE', #18301, 1000.000000000000000 ) ;
#19471=DIRECTION ( 'NONE',  ( 0.000000000000000000, 0.000000000000000000, 1.000000000000000000 ) ) ;
#19473=AXIS2_PLACEMENT_3D ( 'NONE', #4149, #20782, #4386 ) ;
#19478=CARTESIAN_POINT ( 'NONE',  ( -9.302608809283439584, -8.974600000000002353, 5.000000000000079936 ) ) ;
#19484=EDGE_CURVE ( 'NONE', #18054, #19575, #22755, .T. ) ;
#19492=VERTEX_POINT ( 'NONE', #6367 ) ;
#19496=CARTESIAN_POINT ( 'NONE',  ( 47.23681404676619877, -9.000000000000001776, 5.000000000000079936 ) ) ;
#19500=ORIENTED_EDGE ( 'NONE', *, *, #17394, .T. ) ;
#19503=DIRECTION ( 'NONE',  ( 0.3420201433256622181, -0.9396926207859107594, 0.000000000000000000 ) ) ;
#19506=VECTOR ( 'NONE', #9913, 1000.000000000000000 ) ;
#19509=VECTOR ( 'NONE', #6000, 1000.000000000000114 ) ;
#19514=EDGE_CURVE ( 'NONE', #19393, #18250, #13808, .T. ) ;
#19515=ORIENTED_EDGE ( 'NONE', *, *, #8797, .T. ) ;
#19524=LINE ( 'NONE', #13572, #15359 ) ;
#19537=DIRECTION ( 'NONE',  ( 1.000000000000000000, 7.703719777548943412E-32, 0.000000000000000000 ) ) ;
#19538=VECTOR ( 'NONE', #7536, 1000.000000000000000 ) ;
#19539=ORIENTED_EDGE ( 'NONE', *, *, #16152, .T. ) ;
#19541=ORIENTED_EDGE ( 'NONE', *, *, #452, .T. ) ;
#19546=ORIENTED_EDGE ( 'NONE', *, *, #5585, .T. ) ;
#19557=EDGE_CURVE ( 'NONE', #6808, #6494, #22516, .T. ) ;
#19575=VERTEX_POINT ( 'NONE', #10574 ) ;
#19578=EDGE_CURVE ( 'NONE', #17912, #4980, #4789, .T. ) ;
#19581=DIRECTION ( 'NONE',  ( 1.000000000000000000, 7.703719777548943412E-32, 0.000000000000000000 ) ) ;
#19592=ORIENTED_EDGE ( 'NONE', *, *, #2824, .T. ) ;
#19596=VERTEX_POINT ( 'NONE', #12364 ) ;
#19602=CARTESIAN_POINT ( 'NONE',  ( 47.85166990323382663, -9.000000000000005329, 5.000000000000079936 ) ) ;
#19612=ADVANCED_FACE ( 'NONE', ( #19275 ), #21535, .F. ) ;
#19618=CARTESIAN_POINT ( 'NONE',  ( -12.44420145928343935, -8.974600000000002353, 5.000000000000079936 ) ) ;
#19631=DIRECTION ( 'NONE',  ( 1.000000000000000000, 7.703719777548943412E-32, 0.000000000000000000 ) ) ;
#19635=ORIENTED_EDGE ( 'NONE', *, *, #15801, .T. ) ;
#19642=ADVANCED_FACE ( 'NONE', ( #6829 ), #3347, .T. ) ;
#19660=VECTOR ( 'NONE', #7725, 1000.000000000000114 ) ;
#19667=FACE_OUTER_BOUND ( 'NONE', #11126, .T. ) ;
#19668=CARTESIAN_POINT ( 'NONE',  ( 0.7185353092834488864, -8.974600000000002353, 5.000000000000079936 ) ) ;
#19683=VECTOR ( 'NONE', #7014, 1000.000000000000000 ) ;
#19685=AXIS2_PLACEMENT_3D ( 'NONE', #11289, #16546, #3710 ) ;
#19688=ORIENTED_EDGE ( 'NONE', *, *, #7023, .F. ) ;
#19690=LINE ( 'NONE', #4982, #13724 ) ;
#19702=FILL_AREA_STYLE ('',( #12438 ) ) ;
#19704=CARTESIAN_POINT ( 'NONE',  ( 14.11308378033275446, -11.25000000000000355, 5.000000000000079936 ) ) ;
#19707=CARTESIAN_POINT ( 'NONE',  ( 41.55923975928345016, -8.974600000000002353, 5.000000000000079936 ) ) ;
#19719=EDGE_CURVE ( 'NONE', #3801, #9962, #9006, .T. ) ;
#19721=EDGE_LOOP ( 'NONE', ( #22016, #21176, #45, #21450 ) ) ;
#19723=ORIENTED_EDGE ( 'NONE', *, *, #943, .T. ) ;
#19737=EDGE_CURVE ( 'NONE', #16212, #15725, #7675, .T. ) ;
#19739=ORIENTED_EDGE ( 'NONE', *, *, #18587, .T. ) ;
#19741=EDGE_CURVE ( 'NONE', #2131, #22090, #7545, .T. ) ;
#19744=ORIENTED_EDGE ( 'NONE', *, *, #9529, .T. ) ;
#19752=ADVANCED_FACE ( 'NONE', ( #3820 ), #9348, .T. ) ;
#19771=AXIS2_PLACEMENT_3D ( 'NONE', #3270, #5184, #21573 ) ;
#19783=VERTEX_POINT ( 'NONE', #10809 ) ;
#19807=EDGE_CURVE ( 'NONE', #22748, #21720, #9120, .T. ) ;
#19813=FACE_OUTER_BOUND ( 'NONE', #2711, .T. ) ;
#19818=ORIENTED_EDGE ( 'NONE', *, *, #15503, .F. ) ;
#19826=DIRECTION ( 'NONE',  ( -0.3420201433256622181, 0.9396926207859106484, 1.232595164407828100E-31 ) ) ;
#19838=EDGE_LOOP ( 'NONE', ( #21619, #15679, #3158, #2900 ) ) ;
#19841=VECTOR ( 'NONE', #19153, 1000.000000000000114 ) ;
#19854=CARTESIAN_POINT ( 'NONE',  ( 30.70991776966726405, -11.25000000000000355, 10.00000000000008882 ) ) ;
#19855=AXIS2_PLACEMENT_3D ( 'NONE', #586, #20815, #9958 ) ;
#19856=ADVANCED_FACE ( 'NONE', ( #3581 ), #10916, .F. ) ;
#19858=LINE ( 'NONE', #12937, #20048 ) ;
#19865=ORIENTED_EDGE ( 'NONE', *, *, #14816, .F. ) ;
#19878=EDGE_CURVE ( 'NONE', #10792, #3905, #5616, .T. ) ;
#19879=DIRECTION ( 'NONE',  ( 0.000000000000000000, 0.000000000000000000, 1.000000000000000000 ) ) ;
#19884=VECTOR ( 'NONE', #2312, 1000.000000000000000 ) ;
#19886=ADVANCED_FACE ( 'NONE', ( #13533 ), #22481, .T. ) ;
#19893=CARTESIAN_POINT ( 'NONE',  ( -19.99999999999999645, -9.000000000000003553, 5.000000000000079936 ) ) ;
#19895=CARTESIAN_POINT ( 'NONE',  ( -7.878064769667250999, -11.25000000000000355, 5.000000000000079936 ) ) ;
#19914=VECTOR ( 'NONE', #11018, 1000.000000000000000 ) ;
#19922=DIRECTION ( 'NONE',  ( 0.9396926207859107594, -0.3420201433256623291, 3.697785493223492838E-32 ) ) ;
#19928=ORIENTED_EDGE ( 'NONE', *, *, #4797, .T. ) ;
#19932=DIRECTION ( 'NONE',  ( -1.000000000000000000, -7.703719777548943412E-32, 0.000000000000000000 ) ) ;
#19946=DIRECTION ( 'NONE',  ( -1.000000000000000000, -7.703719777548943412E-32, 0.000000000000000000 ) ) ;
#19949=CARTESIAN_POINT ( 'NONE',  ( 45.00000000000000000, -2.399706452296378245, 55.00000000000021316 ) ) ;
#19957=DIRECTION ( 'NONE',  ( -1.000000000000000000, -7.703719777548943412E-32, 0.000000000000000000 ) ) ;
#19964=ORIENTED_EDGE ( 'NONE', *, *, #6308, .T. ) ;
#19973=DIRECTION ( 'NONE',  ( -1.000000000000000000, -7.703719777548943412E-32, 0.000000000000000000 ) ) ;
#19976=ORIENTED_EDGE ( 'NONE', *, *, #5223, .F. ) ;
#19978=CARTESIAN_POINT ( 'NONE',  ( -6.170261003233799890, -9.000000000000003553, 5.000000000000079936 ) ) ;
#19980=DIRECTION ( 'NONE',  ( 1.000000000000000000, 7.703719777548943412E-32, 0.000000000000000000 ) ) ;
#19987=CARTESIAN_POINT ( 'NONE',  ( -18.13102059071655248, -8.974600000000002353, 5.000000000000079936 ) ) ;
#20000=EDGE_CURVE ( 'NONE', #18533, #20897, #2483, .T. ) ;
#20002=ORIENTED_EDGE ( 'NONE', *, *, #13932, .T. ) ;
#20008=VERTEX_POINT ( 'NONE', #4527 ) ;
#20009=VECTOR ( 'NONE', #12121, 1000.000000000000000 ) ;
#20012=EDGE_CURVE ( 'NONE', #16796, #12703, #9704, .T. ) ;
#20021=ADVANCED_FACE ( 'NONE', ( #12671 ), #23287, .F. ) ;
#20032=DIRECTION ( 'NONE',  ( 0.3420201433256622736, 0.9396926207859106484, 0.000000000000000000 ) ) ;
#20036=DIRECTION ( 'NONE',  ( 0.3420201433256622736, 0.9396926207859106484, 0.000000000000000000 ) ) ;
#20040=ADVANCED_FACE ( 'NONE', ( #13775 ), #21034, .F. ) ;
#20045=VECTOR ( 'NONE', #3349, 1000.000000000000114 ) ;
#20046=DIRECTION ( 'NONE',  ( -7.087422195345011518E-32, -1.000000000000000000, -0.000000000000000000 ) ) ;
#20048=VECTOR ( 'NONE', #5252, 1000.000000000000114 ) ;
#20050=CARTESIAN_POINT ( 'NONE',  ( 35.28529930323381336, -9.000000000000001776, 5.000000000000079936 ) ) ;
#20052=FACE_OUTER_BOUND ( 'NONE', #1380, .T. ) ;
#20055=CARTESIAN_POINT ( 'NONE',  ( 4.688305830332750723, -11.25000000000000355, 5.000000000000079936 ) ) ;
#20056=ADVANCED_FACE ( 'NONE', ( #17792 ), #15578, .F. ) ;
#20062=VERTEX_POINT ( 'NONE', #10973 ) ;
#20063=EDGE_CURVE ( 'NONE', #549, #17388, #1718, .T. ) ;
#20067=ORIENTED_EDGE ( 'NONE', *, *, #20605, .T. ) ;
#20070=VECTOR ( 'NONE', #21654, 1000.000000000000000 ) ;
#20071=AXIS2_PLACEMENT_3D ( 'NONE', #4999, #10296, #13765 ) ;
#20075=FACE_OUTER_BOUND ( 'NONE', #11933, .T. ) ;
#20083=VECTOR ( 'NONE', #14902, 1000.000000000000114 ) ;
#20084=DIRECTION ( 'NONE',  ( 0.000000000000000000, 0.000000000000000000, 1.000000000000000000 ) ) ;
#20085=ORIENTED_EDGE ( 'NONE', *, *, #2914, .T. ) ;
#20098=CARTESIAN_POINT ( 'NONE',  ( -2.413812496766191806, -9.000000000000001776, 5.000000000000079936 ) ) ;
#20103=LINE ( 'NONE', #3837, #1477 ) ;
#20107=CARTESIAN_POINT ( 'NONE',  ( -19.99999999999999645, -9.000000000000003553, 5.000000000000079936 ) ) ;
#20121=ORIENTED_EDGE ( 'NONE', *, *, #19719, .F. ) ;
#20157=VECTOR ( 'NONE', #13748, 1000.000000000000114 ) ;
#20158=EDGE_CURVE ( 'NONE', #16343, #13221, #14218, .T. ) ;
#20162=CARTESIAN_POINT ( 'NONE',  ( 2.435583919667260400, -11.25000000000000355, 10.00000000000008882 ) ) ;
#20167=DIRECTION ( 'NONE',  ( 1.000000000000000000, 7.703719777548943412E-32, 0.000000000000000000 ) ) ;
#20169=ADVANCED_FACE ( 'NONE', ( #3290 ), #10632, .F. ) ;
#20171=CARTESIAN_POINT ( 'NONE',  ( -6.989194030332740226, -11.25000000000000355, 5.000000000000079936 ) ) ;
#20173=LINE ( 'NONE', #3897, #2674 ) ;
#20174=LINE ( 'NONE', #3899, #12207 ) ;
#20178=ORIENTED_EDGE ( 'NONE', *, *, #8101, .F. ) ;
#20196=VECTOR ( 'NONE', #9323, 1000.000000000000000 ) ;
#20198=LINE ( 'NONE', #18186, #19914 ) ;
#20200=CARTESIAN_POINT ( 'NONE',  ( 21.28513981966725765, -11.25000000000000355, 5.000000000000079936 ) ) ;
#20215=ORIENTED_EDGE ( 'NONE', *, *, #22970, .F. ) ;
#20217=DIRECTION ( 'NONE',  ( 0.000000000000000000, 0.000000000000000000, 1.000000000000000000 ) ) ;
#20222=CARTESIAN_POINT ( 'NONE',  ( -12.79329400524661331, -6.376973530802017898, 10.00000000000008882 ) ) ;
#20229=EDGE_CURVE ( 'NONE', #10792, #18482, #22424, .T. ) ;
#20238=DIRECTION ( 'NONE',  ( -0.9396926207859107594, -0.3420201433256623291, 1.540743955509804830E-32 ) ) ;
#20255=VECTOR ( 'NONE', #22898, 1000.000000000000000 ) ;
#20266=AXIS2_PLACEMENT_3D ( 'NONE', #14756, #6104, #5627 ) ;
#20279=DIRECTION ( 'NONE',  ( 0.9396926207859107594, -0.3420201433256623291, 3.697785493223492838E-32 ) ) ;
#20280=VERTEX_POINT ( 'NONE', #5801 ) ;
#20282=CARTESIAN_POINT ( 'NONE',  ( 17.25467643033275067, -11.25000000000000355, 10.00000000000008882 ) ) ;
#20284=VECTOR ( 'NONE', #8519, 1000.000000000000000 ) ;
#20295=LINE ( 'NONE', #5705, #2464 ) ;
#20303=ORIENTED_EDGE ( 'NONE', *, *, #20229, .F. ) ;
#20307=ADVANCED_FACE ( 'NONE', ( #14690 ), #9410, .F. ) ;
#20321=CARTESIAN_POINT ( 'NONE',  ( -19.99999999999999645, -15.00000000000001954, 10.00000000000008882 ) ) ;
#20331=ORIENTED_EDGE ( 'NONE', *, *, #12124, .T. ) ;
#20334=DIRECTION ( 'NONE',  ( -1.000000000000000000, -7.703719777548943412E-32, 0.000000000000000000 ) ) ;
#20336=ADVANCED_FACE ( 'NONE', ( #16700 ), #11090, .F. ) ;
#20339=DIRECTION ( 'NONE',  ( -1.000000000000000000, -7.703719777548943412E-32, 0.000000000000000000 ) ) ;
#20343=CIRCLE ( 'NONE', #80, 5.000000000000011546 ) ;
#20359=ORIENTED_EDGE ( 'NONE', *, *, #17861, .F. ) ;
#20363=VERTEX_POINT ( 'NONE', #3996 ) ;
#20366=VECTOR ( 'NONE', #15127, 1000.000000000000000 ) ;
#20388=VECTOR ( 'NONE', #10913, 1000.000000000000114 ) ;
#20389=CARTESIAN_POINT ( 'NONE',  ( 118.3095189484530181, -15.00000000000001954, 10.00000000000008882 ) ) ;
#20394=ORIENTED_EDGE ( 'NONE', *, *, #10101, .T. ) ;
#20401=LINE ( 'NONE', #16596, #12790 ) ;
#20407=FACE_OUTER_BOUND ( 'NONE', #18406, .T. ) ;
#20415=ORIENTED_EDGE ( 'NONE', *, *, #18619, .F. ) ;
#20427=VECTOR ( 'NONE', #595, 1000.000000000000114 ) ;
#20431=EDGE_CURVE ( 'NONE', #23005, #17845, #23254, .T. ) ;
#20436=PLANE ( 'NONE',  #734 ) ;
#20440=ORIENTED_EDGE ( 'NONE', *, *, #13406, .F. ) ;
#20451=DIRECTION ( 'NONE',  ( 0.3420201433256622181, -0.9396926207859107594, 0.000000000000000000 ) ) ;
#20469=PLANE ( 'NONE',  #15523 ) ;
#20479=ORIENTED_EDGE ( 'NONE', *, *, #10277, .F. ) ;
#20481=VERTEX_POINT ( 'NONE', #14056 ) ;
#20485=EDGE_LOOP ( 'NONE', ( #21974, #17272, #18245, #10425 ) ) ;
#20496=DIRECTION ( 'NONE',  ( -7.087422195345011518E-32, -1.000000000000000000, -0.000000000000000000 ) ) ;
#20505=ORIENTED_EDGE ( 'NONE', *, *, #5223, .T. ) ;
#20517=AXIS2_PLACEMENT_3D ( 'NONE', #3047, #19922, #10395 ) ;
#20522=VECTOR ( 'NONE', #964, 1000.000000000000114 ) ;
#20527=ADVANCED_FACE ( 'NONE', ( #11189 ), #5894, .T. ) ;
#20536=ORIENTED_EDGE ( 'NONE', *, *, #16539, .F. ) ;
#20538=VECTOR ( 'NONE', #16774, 1000.000000000000114 ) ;
#20542=ORIENTED_EDGE ( 'NONE', *, *, #546, .F. ) ;
#20544=ORIENTED_EDGE ( 'NONE', *, *, #13944, .F. ) ;
#20550=CARTESIAN_POINT ( 'NONE',  ( 43.27628836966725601, -11.25000000000000355, 5.000000000000079936 ) ) ;
#20553=VECTOR ( 'NONE', #22227, 1000.000000000000000 ) ;
#20564=DIRECTION ( 'NONE',  ( -1.000000000000000000, -7.703719777548943412E-32, 0.000000000000000000 ) ) ;
#20574=ADVANCED_FACE ( 'NONE', ( #24 ), #15137, .F. ) ;
#20577=DIRECTION ( 'NONE',  ( -0.3420201433256622181, 0.9396926207859106484, 1.232595164407828100E-31 ) ) ;
#20582=PLANE ( 'NONE',  #15981 ) ;
#20594=CARTESIAN_POINT ( 'NONE',  ( -15.59503895323380362, -9.000000000000003553, 5.000000000000079936 ) ) ;
#20603=LINE ( 'NONE', #15490, #12498 ) ;
#20605=EDGE_CURVE ( 'NONE', #12674, #1126, #9407, .T. ) ;
#20607=ORIENTED_EDGE ( 'NONE', *, *, #22400, .F. ) ;
#20620=DIRECTION ( 'NONE',  ( 7.087422195345011518E-32, 1.000000000000000000, -0.000000000000000000 ) ) ;
#20625=AXIS2_PLACEMENT_3D ( 'NONE', #9546, #14948, #5933 ) ;
#20633=CARTESIAN_POINT ( 'NONE',  ( 16.42649855928345204, -8.974600000000002353, 5.000000000000079936 ) ) ;
#20634=ORIENTED_EDGE ( 'NONE', *, *, #17317, .F. ) ;
#20638=EDGE_CURVE ( 'NONE', #2345, #12921, #3854, .T. ) ;
#20642=EDGE_CURVE ( 'NONE', #18509, #13840, #248, .T. ) ;
#20652=VECTOR ( 'NONE', #6512, 1000.000000000000000 ) ;
#20656=CARTESIAN_POINT ( 'NONE',  ( 18.14354716966726144, -11.25000000000000355, 5.000000000000079936 ) ) ;
#20659=ORIENTED_EDGE ( 'NONE', *, *, #5825, .T. ) ;
#20663=ORIENTED_EDGE ( 'NONE', *, *, #974, .T. ) ;
#20670=EDGE_CURVE ( 'NONE', #14446, #15725, #2870, .T. ) ;
#20674=FACE_OUTER_BOUND ( 'NONE', #19838, .T. ) ;
#20681=VECTOR ( 'NONE', #2857, 1000.000000000000000 ) ;
#20684=EDGE_LOOP ( 'NONE', ( #7408, #5886, #22094, #14117 ) ) ;
#20688=CARTESIAN_POINT ( 'NONE',  ( 45.00000000000000000, -10.00000000000001599, 34.11836509645782201 ) ) ;
#20689=ORIENTED_EDGE ( 'NONE', *, *, #10123, .F. ) ;
#20723=LINE ( 'NONE', #22644, #983 ) ;
#20724=ORIENTED_EDGE ( 'NONE', *, *, #5858, .F. ) ;
#20731=DIRECTION ( 'NONE',  ( 1.000000000000000000, 7.703719777548943412E-32, 0.000000000000000000 ) ) ;
#20734=EDGE_CURVE ( 'NONE', #14420, #14717, #17275, .T. ) ;
#20739=DIRECTION ( 'NONE',  ( 0.000000000000000000, 0.000000000000000000, 1.000000000000000000 ) ) ;
#20751=CARTESIAN_POINT ( 'NONE',  ( -19.99999999999999645, -9.000000000000003553, 10.00000000000008882 ) ) ;
#20754=LINE ( 'NONE', #6405, #4872 ) ;
#20755=CARTESIAN_POINT ( 'NONE',  ( 29.82104703033275328, -11.25000000000000355, 5.000000000000079936 ) ) ;
#20758=CARTESIAN_POINT ( 'NONE',  ( 47.24605889071655440, -8.974600000000002353, 5.000000000000079936 ) ) ;
#20765=EDGE_CURVE ( 'NONE', #476, #10312, #10186, .T. ) ;
#20771=DIRECTION ( 'NONE',  ( 0.000000000000000000, 0.000000000000000000, 1.000000000000000000 ) ) ;
#20779=CLOSED_SHELL ( 'NONE', ( #14517, #387, #10037, #18282, #9214, #16190, #22222, #9247, #3197, #12487, #19886, #17007, #20336, #19218, #7715, #21316, #20040, #22252, #9597, #1935, #10007, #4979, #7311, #23258, #5804, #20926, #16885, #9421, #1575, #3647, #19642, #10890, #13466, #15234, #20527, #11498, #2037, #16279, #18992, #15826, #19752, #18154, #16949, #3266, #2793, #14611, #9965, #275, #17151, #21832, #11125, #11625, #2955, #11195, #20021, #5129, #20169, #8105, #6577, #13177, #10868, #14008, #18331, #1068, #22703, #15247, #5095, #13018, #13025, #7195, #20056, #10261, #14102, #4673, #7569, #19282, #1302, #3128, #19612, #4575, #18196, #12293, #22404, #20574, #3268, #4064, #8930, #13715, #1707, #7640, #9558, #7923, #19856, #5931, #17833, #17682, #20307, #11046, #22352, #7916, #13491, #14836, #13744, #5270, #18436, #5425, #5619, #4701, #8266, #16354, #7369, #14831, #23302, #879 ) ) ;
#20780=LINE ( 'NONE', #4384, #22069 ) ;
#20782=DIRECTION ( 'NONE',  ( 1.000000000000000000, 7.703719777548943412E-32, 0.000000000000000000 ) ) ;
#20787=VERTEX_POINT ( 'NONE', #10218 ) ;
#20791=EDGE_CURVE ( 'NONE', #4634, #7447, #9985, .T. ) ;
#20795=CARTESIAN_POINT ( 'NONE',  ( 50.00000000000000000, 10.00000000000001599, 34.11836509645781490 ) ) ;
#20796=ORIENTED_EDGE ( 'NONE', *, *, #18195, .F. ) ;
#20797=LINE ( 'NONE', #4522, #6521 ) ;
#20801=EDGE_CURVE ( 'NONE', #1016, #5492, #20603, .T. ) ;
#20802=ORIENTED_EDGE ( 'NONE', *, *, #17080, .T. ) ;
#20805=CARTESIAN_POINT ( 'NONE',  ( 50.00000000000000000, -10.03966385473554013, 10.00000000000008882 ) ) ;
#20808=FACE_OUTER_BOUND ( 'NONE', #14939, .T. ) ;
#20811=VECTOR ( 'NONE', #9648, 1000.000000000000000 ) ;
#20814=ORIENTED_EDGE ( 'NONE', *, *, #5557, .F. ) ;
#20815=DIRECTION ( 'NONE',  ( -1.000000000000000000, -7.703719777548943412E-32, 0.000000000000000000 ) ) ;
#20817=ORIENTED_EDGE ( 'NONE', *, *, #15801, .F. ) ;
#20834=ORIENTED_EDGE ( 'NONE', *, *, #9095, .T. ) ;
#20847=DIRECTION ( 'NONE',  ( 0.3420201433256622736, -0.9396926207859106484, -1.232595164407828100E-31 ) ) ;
#20851=LINE ( 'NONE', #13830, #15494 ) ;
#20862=ORIENTED_EDGE ( 'NONE', *, *, #15438, .T. ) ;
#20869=CARTESIAN_POINT ( 'NONE',  ( 10.15255810323380992, -9.000000000000003553, 5.000000000000079936 ) ) ;
#20871=EDGE_CURVE ( 'NONE', #7229, #15755, #20723, .T. ) ;
#20885=CARTESIAN_POINT ( 'NONE',  ( 41.55923975928345016, -8.974600000000002353, 5.000000000000079936 ) ) ;
#20897=VERTEX_POINT ( 'NONE', #1667 ) ;
#20900=LINE ( 'NONE', #10173, #6112 ) ;
#20902=DIRECTION ( 'NONE',  ( -0.9396926207859107594, -0.3420201433256623291, 1.540743955509804830E-32 ) ) ;
#20904=PLANE ( 'NONE',  #20071 ) ;
#20926=ADVANCED_FACE ( 'NONE', ( #8641 ), #21421, .T. ) ;
#20931=CARTESIAN_POINT ( 'NONE',  ( -15.58579410928343911, -8.974600000000002353, 10.00000000000008882 ) ) ;
#20935=LINE ( 'NONE', #16906, #17024 ) ;
#20941=DIRECTION ( 'NONE',  ( -1.000000000000000000, -7.703719777548943412E-32, 0.000000000000000000 ) ) ;
#20944=DIRECTION ( 'NONE',  ( 0.3420201433256622181, 0.9396926207859107594, -6.162975822039141593E-32 ) ) ;
#20948=CARTESIAN_POINT ( 'NONE',  ( -19.99999999999999645, -9.000000000000003553, 5.000000000000079936 ) ) ;
#20950=VECTOR ( 'NONE', #868, 1000.000000000000000 ) ;
#20956=EDGE_CURVE ( 'NONE', #19596, #4473, #21626, .T. ) ;
#20970=ORIENTED_EDGE ( 'NONE', *, *, #5419, .F. ) ;
#20977=CARTESIAN_POINT ( 'NONE',  ( -10.13078668033273999, -11.25000000000000355, 10.00000000000008882 ) ) ;
#20990=VECTOR ( 'NONE', #23569, 1000.000000000000000 ) ;
#20998=DIRECTION ( 'NONE',  ( 0.000000000000000000, 0.000000000000000000, 1.000000000000000000 ) ) ;
#21012=VERTEX_POINT ( 'NONE', #16182 ) ;
#21013=LINE ( 'NONE', #8482, #17191 ) ;
#21030=PLANE ( 'NONE',  #15553 ) ;
#21031=FACE_OUTER_BOUND ( 'NONE', #920, .T. ) ;
#21034=PLANE ( 'NONE',  #3632 ) ;
#21039=PLANE ( 'NONE',  #4109 ) ;
#21049=AXIS2_PLACEMENT_3D ( 'NONE', #205, #9108, #1996 ) ;
#21060=PLANE ( 'NONE',  #4808 ) ;
#21069=EDGE_CURVE ( 'NONE', #20008, #16796, #18546, .T. ) ;
#21099=VERTEX_POINT ( 'NONE', #4059 ) ;
#21104=LINE ( 'NONE', #10254, #14129 ) ;
#21121=SHAPE_REPRESENTATION_RELATIONSHIP ( 'NONE' , 'NONE' ,  #18175, #449 ) ;
#21147=DIRECTION ( 'NONE',  ( 0.000000000000000000, 0.000000000000000000, 1.000000000000000000 ) ) ;
#21157=LINE ( 'NONE', #21270, #16818 ) ;
#21163=DIRECTION ( 'NONE',  ( 0.000000000000000000, 0.000000000000000000, 1.000000000000000000 ) ) ;
#21167=DIRECTION ( 'NONE',  ( 0.000000000000000000, 0.000000000000000000, 1.000000000000000000 ) ) ;
#21176=ORIENTED_EDGE ( 'NONE', *, *, #9670, .F. ) ;
#21179=DIRECTION ( 'NONE',  ( 7.087422195345011518E-32, 1.000000000000000000, -0.000000000000000000 ) ) ;
#21188=AXIS2_PLACEMENT_3D ( 'NONE', #18953, #19300, #12037 ) ;
#21208=CARTESIAN_POINT ( 'NONE',  ( -11.83859044676619199, -9.000000000000003553, 10.00000000000008882 ) ) ;
#21212=CARTESIAN_POINT ( 'NONE',  ( 5.577176569667260608, -11.25000000000000355, 5.000000000000079936 ) ) ;
#21218=DIRECTION ( 'NONE',  ( 0.000000000000000000, 0.000000000000000000, -1.000000000000000000 ) ) ;
#21224=VECTOR ( 'NONE', #5175, 1000.000000000000000 ) ;
#21230=CARTESIAN_POINT ( 'NONE',  ( 4.688305830332750723, -11.25000000000000355, 10.00000000000008882 ) ) ;
#21235=VERTEX_POINT ( 'NONE', #18796 ) ;
#21242=DIRECTION ( 'NONE',  ( 1.000000000000000000, 7.703719777548943412E-32, 0.000000000000000000 ) ) ;
#21243=ORIENTED_EDGE ( 'NONE', *, *, #10275, .F. ) ;
#21244=LINE ( 'NONE', #21481, #10709 ) ;
#21257=DIRECTION ( 'NONE',  ( 1.000000000000000000, 7.703719777548943412E-32, 0.000000000000000000 ) ) ;
#21261=DIRECTION ( 'NONE',  ( 0.3420201433256622181, 0.9396926207859107594, -6.162975822039141593E-32 ) ) ;
#21264=ORIENTED_EDGE ( 'NONE', *, *, #19180, .F. ) ;
#21269=VECTOR ( 'NONE', #10506, 1000.000000000000114 ) ;
#21270=CARTESIAN_POINT ( 'NONE',  ( 30.70991776966726405, -11.25000000000000355, 5.000000000000079936 ) ) ;
#21273=ORIENTED_EDGE ( 'NONE', *, *, #10428, .F. ) ;
#21288=EDGE_CURVE ( 'NONE', #15099, #18435, #15292, .T. ) ;
#21290=ORIENTED_EDGE ( 'NONE', *, *, #6472, .T. ) ;
#21308=VECTOR ( 'NONE', #11010, 1000.000000000000000 ) ;
#21315=ORIENTED_EDGE ( 'NONE', *, *, #20063, .F. ) ;
#21316=ADVANCED_FACE ( 'NONE', ( #22616, #22368, #5979, #20808 ), #4415, .T. ) ;
#21318=DIRECTION ( 'NONE',  ( 0.000000000000000000, 0.000000000000000000, 1.000000000000000000 ) ) ;
#21319=ORIENTED_EDGE ( 'NONE', *, *, #7323, .F. ) ;
#21357=ORIENTED_EDGE ( 'NONE', *, *, #14106, .F. ) ;
#21358=VECTOR ( 'NONE', #3695, 1000.000000000000114 ) ;
#21366=VERTEX_POINT ( 'NONE', #19602 ) ;
#21372=DIRECTION ( 'NONE',  ( 0.3420201433256622181, 0.9396926207859107594, -6.162975822039141593E-32 ) ) ;
#21390=PLANE ( 'NONE',  #15233 ) ;
#21392=ORIENTED_EDGE ( 'NONE', *, *, #16152, .F. ) ;
#21400=DIRECTION ( 'NONE',  ( 0.000000000000000000, 0.000000000000000000, 1.000000000000000000 ) ) ;
#21404=CARTESIAN_POINT ( 'NONE',  ( 16.43574340323381122, -9.000000000000001776, 5.000000000000079936 ) ) ;
#21408=LINE ( 'NONE', #12116, #13978 ) ;
#21410=VECTOR ( 'NONE', #18599, 1000.000000000000000 ) ;
#21416=ORIENTED_EDGE ( 'NONE', *, *, #10164, .T. ) ;
#21417=DIRECTION ( 'NONE',  ( 0.000000000000000000, 0.000000000000000000, -1.000000000000000000 ) ) ;
#21418=DIRECTION ( 'NONE',  ( 0.000000000000000000, 0.000000000000000000, -1.000000000000000000 ) ) ;
#21420=ORIENTED_EDGE ( 'NONE', *, *, #14104, .T. ) ;
#21421=PLANE ( 'NONE',  #6352 ) ;
#21427=LINE ( 'NONE', #8425, #2936 ) ;
#21430=EDGE_CURVE ( 'NONE', #5492, #22748, #23081, .T. ) ;
#21435=LINE ( 'NONE', #10594, #3415 ) ;
#21438=FACE_OUTER_BOUND ( 'NONE', #22403, .T. ) ;
#21441=LINE ( 'NONE', #8666, #17399 ) ;
#21450=ORIENTED_EDGE ( 'NONE', *, *, #2620, .T. ) ;
#21456=EDGE_CURVE ( 'NONE', #6956, #17853, #8729, .T. ) ;
#21457=CARTESIAN_POINT ( 'NONE',  ( 28.39650299071657003, -8.974600000000002353, 10.00000000000008882 ) ) ;
#21465=DIRECTION ( 'NONE',  ( -1.000000000000000000, -7.703719777548943412E-32, 0.000000000000000000 ) ) ;
#21477=VERTEX_POINT ( 'NONE', #13894 ) ;
#21479=FACE_OUTER_BOUND ( 'NONE', #13945, .T. ) ;
#21480=ORIENTED_EDGE ( 'NONE', *, *, #10305, .T. ) ;
#21481=CARTESIAN_POINT ( 'NONE',  ( 34.67968829071656245, -8.974600000000002353, 5.000000000000079936 ) ) ;
#21490=DIRECTION ( 'NONE',  ( 0.000000000000000000, 0.000000000000000000, 1.000000000000000000 ) ) ;
#21497=LINE ( 'NONE', #5108, #4412 ) ;
#21510=EDGE_LOOP ( 'NONE', ( #17531, #6587, #10812, #3781 ) ) ;
#21516=EDGE_CURVE ( 'NONE', #16343, #3172, #21749, .T. ) ;
#21519=APPLICATION_CONTEXT ( 'automotive_design' ) ;
#21526=EDGE_CURVE ( 'NONE', #5147, #12674, #22219, .T. ) ;
#21528=CARTESIAN_POINT ( 'NONE',  ( 24.42673246966726452, -11.25000000000000355, 5.000000000000079936 ) ) ;
#21534=VERTEX_POINT ( 'NONE', #7170 ) ;
#21535=PLANE ( 'NONE',  #14761 ) ;
#21540=ORIENTED_EDGE ( 'NONE', *, *, #12057, .F. ) ;
#21541=DIRECTION ( 'NONE',  ( -7.087422195345011518E-32, -1.000000000000000000, 0.000000000000000000 ) ) ;
#21556=CARTESIAN_POINT ( 'NONE',  ( 18.14354716966726144, -11.25000000000000355, 10.00000000000008882 ) ) ;
#21559=EDGE_LOOP ( 'NONE', ( #22899, #5807 ) ) ;
#21566=ORIENTED_EDGE ( 'NONE', *, *, #7060, .T. ) ;
#21573=DIRECTION ( 'NONE',  ( 0.000000000000000000, 0.000000000000000000, -1.000000000000000000 ) ) ;
#21596=EDGE_LOOP ( 'NONE', ( #5649, #6237, #20607, #23466 ) ) ;
#21602=CARTESIAN_POINT ( 'NONE',  ( 8.718769219667262149, -11.25000000000000355, 5.000000000000079936 ) ) ;
#21606=VECTOR ( 'NONE', #10097, 1000.000000000000000 ) ;
#21619=ORIENTED_EDGE ( 'NONE', *, *, #2470, .T. ) ;
#21626=CIRCLE ( 'NONE', #7124, 2.500000000000007550 ) ;
#21628=ORIENTED_EDGE ( 'NONE', *, *, #119, .F. ) ;
#21629=CARTESIAN_POINT ( 'NONE',  ( 44.00000000000000711, -9.261618637464055226, 10.00000000000008882 ) ) ;
#21630=VERTEX_POINT ( 'NONE', #7648 ) ;
#21634=EDGE_CURVE ( 'NONE', #16343, #9962, #12809, .T. ) ;
#21641=LINE ( 'NONE', #5372, #1871 ) ;
#21654=DIRECTION ( 'NONE',  ( 0.000000000000000000, 0.000000000000000000, -1.000000000000000000 ) ) ;
#21664=EDGE_CURVE ( 'NONE', #22158, #4844, #77, .T. ) ;
#21666=EDGE_CURVE ( 'NONE', #7447, #129, #23482, .T. ) ;
#21669=PLANE ( 'NONE',  #11777 ) ;
#21679=DIRECTION ( 'NONE',  ( -1.000000000000000000, -7.703719777548943412E-32, 0.000000000000000000 ) ) ;
#21680=EDGE_LOOP ( 'NONE', ( #12552, #21392, #4766, #14049 ) ) ;
#21690=FACE_OUTER_BOUND ( 'NONE', #3166, .T. ) ;
#21708=ORIENTED_EDGE ( 'NONE', *, *, #524, .F. ) ;
#21709=CARTESIAN_POINT ( 'NONE',  ( 0.7277801532338118440, -9.000000000000003553, 5.000000000000079936 ) ) ;
#21717=ORIENTED_EDGE ( 'NONE', *, *, #14061, .T. ) ;
#21718=VECTOR ( 'NONE', #8297, 1000.000000000000000 ) ;
#21720=VERTEX_POINT ( 'NONE', #11364 ) ;
#21721=DIRECTION ( 'NONE',  ( -1.000000000000000000, -7.703719777548943412E-32, 0.000000000000000000 ) ) ;
#21723=VECTOR ( 'NONE', #11357, 1000.000000000000000 ) ;
#21726=VERTEX_POINT ( 'NONE', #11842 ) ;
#21731=EDGE_CURVE ( 'NONE', #10312, #4233, #13157, .T. ) ;
#21736=LINE ( 'NONE', #5348, #9020 ) ;
#21737=PLANE ( 'NONE',  #6729 ) ;
#21748=EDGE_LOOP ( 'NONE', ( #6634, #1647, #3665, #13074 ) ) ;
#21749=LINE ( 'NONE', #3669, #9541 ) ;
#21756=LINE ( 'NONE', #18178, #2662 ) ;
#21762=DIRECTION ( 'NONE',  ( 7.087422195345011518E-32, 1.000000000000000000, 0.000000000000000000 ) ) ;
#21763=EDGE_CURVE ( 'NONE', #18607, #17296, #22457, .T. ) ;
#21770=DIRECTION ( 'NONE',  ( 1.000000000000000000, 7.703719777548943412E-32, 0.000000000000000000 ) ) ;
#21771=ORIENTED_EDGE ( 'NONE', *, *, #22860, .F. ) ;
#21778=DIRECTION ( 'NONE',  ( 0.3420201433256622181, 0.9396926207859107594, -6.162975822039141593E-32 ) ) ;
#21779=PLANE ( 'NONE',  #9918 ) ;
#21782=ORIENTED_EDGE ( 'NONE', *, *, #9360, .T. ) ;
#21784=VERTEX_POINT ( 'NONE', #6315 ) ;
#21785=VERTEX_POINT ( 'NONE', #13276 ) ;
#21798=DIRECTION ( 'NONE',  ( -1.000000000000000000, -7.703719777548943412E-32, 0.000000000000000000 ) ) ;
#21808=EDGE_CURVE ( 'NONE', #10807, #22879, #9931, .T. ) ;
#21816=ORIENTED_EDGE ( 'NONE', *, *, #16088, .T. ) ;
#21817=AXIS2_PLACEMENT_3D ( 'NONE', #22764, #8646, #4921 ) ;
#21827=CIRCLE ( 'NONE', #16111, 1.000000000000002665 ) ;
#21828=PLANE ( 'NONE',  #11412 ) ;
#21829=EDGE_CURVE ( 'NONE', #4570, #21012, #11493, .T. ) ;
#21832=ADVANCED_FACE ( 'NONE', ( #13983 ), #12194, .F. ) ;
#21850=DIRECTION ( 'NONE',  ( -0.9396926207859107594, -0.3420201433256623291, 1.540743955509804830E-32 ) ) ;
#21863=ORIENTED_EDGE ( 'NONE', *, *, #11733, .F. ) ;
#21867=VERTEX_POINT ( 'NONE', #14225 ) ;
#21873=CARTESIAN_POINT ( 'NONE',  ( -19.99999999999999645, -9.000000000000003553, 10.00000000000008882 ) ) ;
#21880=PLANE ( 'NONE',  #21049 ) ;
#21890=CARTESIAN_POINT ( 'NONE',  ( -3.019423509283438722, -8.974600000000002353, 5.000000000000079936 ) ) ;
#21900=CARTESIAN_POINT ( 'NONE',  ( 46.41788101966725577, -11.25000000000000355, 10.00000000000008882 ) ) ;
#21901=CARTESIAN_POINT ( 'NONE',  ( 11.86036186966726191, -11.25000000000000355, 10.00000000000008882 ) ) ;
#21919=DIRECTION ( 'NONE',  ( 1.000000000000000000, 7.703719777548943412E-32, 0.000000000000000000 ) ) ;
#21922=EDGE_CURVE ( 'NONE', #476, #22239, #21013, .T. ) ;
#21924=ORIENTED_EDGE ( 'NONE', *, *, #19443, .F. ) ;
#21928=EDGE_CURVE ( 'NONE', #16967, #18422, #21244, .T. ) ;
#21934=CARTESIAN_POINT ( 'NONE',  ( -19.99999999999999645, -9.000000000000003553, 10.00000000000008882 ) ) ;
#21940=ORIENTED_EDGE ( 'NONE', *, *, #23679, .F. ) ;
#21946=DIRECTION ( 'NONE',  ( 0.3420201433256622736, 0.9396926207859106484, 0.000000000000000000 ) ) ;
#21954=CARTESIAN_POINT ( 'NONE',  ( 15.00195451966726523, -11.25000000000000355, 10.00000000000008882 ) ) ;
#21958=CARTESIAN_POINT ( 'NONE',  ( -18.13102059071655248, -8.974600000000002353, 5.000000000000079936 ) ) ;
#21959=VECTOR ( 'NONE', #8757, 1000.000000000000000 ) ;
#21968=CARTESIAN_POINT ( 'NONE',  ( -11.01965741966725076, -11.25000000000000355, 5.000000000000079936 ) ) ;
#21972=CARTESIAN_POINT ( 'NONE',  ( -19.99999999999999645, -9.000000000000003553, 5.000000000000079936 ) ) ;
#21973=ORIENTED_EDGE ( 'NONE', *, *, #7765, .T. ) ;
#21974=ORIENTED_EDGE ( 'NONE', *, *, #15774, .T. ) ;
#21983=AXIS2_PLACEMENT_3D ( 'NONE', #11376, #15207, #6082 ) ;
#21987=LINE ( 'NONE', #22463, #284 ) ;
#21989=VERTEX_POINT ( 'NONE', #18035 ) ;
#21997=LINE ( 'NONE', #3683, #7300 ) ;
#22006=CARTESIAN_POINT ( 'NONE',  ( -6.161016159283438931, -8.974600000000002353, 10.00000000000008882 ) ) ;
#22012=CARTESIAN_POINT ( 'NONE',  ( 22.71892870323381075, -9.000000000000005329, 10.00000000000008882 ) ) ;
#22016=ORIENTED_EDGE ( 'NONE', *, *, #5765, .T. ) ;
#22022=EDGE_CURVE ( 'NONE', #13240, #3850, #8954, .T. ) ;
#22026=VERTEX_POINT ( 'NONE', #9066 ) ;
#22032=EDGE_CURVE ( 'NONE', #5149, #22090, #9302, .T. ) ;
#22034=ORIENTED_EDGE ( 'NONE', *, *, #22228, .F. ) ;
#22035=ORIENTED_EDGE ( 'NONE', *, *, #11284, .T. ) ;
#22049=VECTOR ( 'NONE', #2374, 1000.000000000000000 ) ;
#22059=ORIENTED_EDGE ( 'NONE', *, *, #8964, .T. ) ;
#22065=LINE ( 'NONE', #1843, #14441 ) ;
#22069=VECTOR ( 'NONE', #11491, 1000.000000000000114 ) ;
#22072=CARTESIAN_POINT ( 'NONE',  ( -10.13078668033273999, -11.25000000000000355, 10.00000000000008882 ) ) ;
#22075=EDGE_CURVE ( 'NONE', #1035, #1856, #12507, .T. ) ;
#22080=VECTOR ( 'NONE', #12464, 1000.000000000000000 ) ;
#22088=VECTOR ( 'NONE', #21242, 1000.000000000000000 ) ;
#22090=VERTEX_POINT ( 'NONE', #6974 ) ;
#22094=ORIENTED_EDGE ( 'NONE', *, *, #18149, .F. ) ;
#22116=LINE ( 'NONE', #5738, #16666 ) ;
#22117=CARTESIAN_POINT ( 'NONE',  ( 45.00000000000000000, -2.399706452296352932, 60.00000000000021316 ) ) ;
#22121=EDGE_LOOP ( 'NONE', ( #21924, #16492, #3090, #18524 ) ) ;
#22122=CIRCLE ( 'NONE', #13735, 2.500000000000007550 ) ;
#22125=CARTESIAN_POINT ( 'NONE',  ( -19.99999999999999645, -9.000000000000003553, 10.00000000000008882 ) ) ;
#22127=ORIENTED_EDGE ( 'NONE', *, *, #15954, .T. ) ;
#22132=VECTOR ( 'NONE', #1249, 1000.000000000000114 ) ;
#22138=CIRCLE ( 'NONE', #7645, 5.000000000000011546 ) ;
#22154=EDGE_LOOP ( 'NONE', ( #6271, #4572, #19541, #19865 ) ) ;
#22158=VERTEX_POINT ( 'NONE', #3248 ) ;
#22178=CARTESIAN_POINT ( 'NONE',  ( -0.7060087303327398089, -11.25000000000000355, 5.000000000000079936 ) ) ;
#22182=CARTESIAN_POINT ( 'NONE',  ( 21.28513981966725765, -11.25000000000000355, 5.000000000000079936 ) ) ;
#22185=VECTOR ( 'NONE', #10572, 1000.000000000000000 ) ;
#22188=VERTEX_POINT ( 'NONE', #13939 ) ;
#22199=EDGE_CURVE ( 'NONE', #22527, #18533, #21435, .T. ) ;
#22200=PLANE ( 'NONE',  #513 ) ;
#22207=CARTESIAN_POINT ( 'NONE',  ( 25.86052135323381407, -9.000000000000001776, 5.000000000000079936 ) ) ;
#22219=LINE ( 'NONE', #14607, #20196 ) ;
#22222=ADVANCED_FACE ( 'NONE', ( #3773 ), #17924, .T. ) ;
#22226=DIRECTION ( 'NONE',  ( 0.000000000000000000, 0.000000000000000000, 1.000000000000000000 ) ) ;
#22227=DIRECTION ( 'NONE',  ( 0.000000000000000000, 0.000000000000000000, 1.000000000000000000 ) ) ;
#22228=EDGE_CURVE ( 'NONE', #14446, #16796, #7398, .T. ) ;
#22231=EDGE_CURVE ( 'NONE', #8738, #3905, #9078, .T. ) ;
#22234=CARTESIAN_POINT ( 'NONE',  ( -14.98942794071655271, -8.974600000000002353, 5.000000000000079936 ) ) ;
#22239=VERTEX_POINT ( 'NONE', #12797 ) ;
#22240=CARTESIAN_POINT ( 'NONE',  ( 45.00000000000000000, -9.796556200126357083, 5.000000000000079936 ) ) ;
#22252=ADVANCED_FACE ( 'NONE', ( #1853 ), #3431, .F. ) ;
#22275=VERTEX_POINT ( 'NONE', #20050 ) ;
#22288=MANIFOLD_SOLID_BREP ( 'Fillet1', #20779 ) ;
#22297=CARTESIAN_POINT ( 'NONE',  ( 45.00000000000000000, 2.399706452296377801, 55.00000000000021316 ) ) ;
#22306=DIRECTION ( 'NONE',  ( 7.200064461366508930E-32, 1.000000000000000000, 5.754033390038003495E-16 ) ) ;
#22334=EDGE_CURVE ( 'NONE', #549, #2702, #13387, .T. ) ;
#22341=AXIS2_PLACEMENT_3D ( 'NONE', #11572, #15398, #22900 ) ;
#22352=ADVANCED_FACE ( 'NONE', ( #20407 ), #11596, .F. ) ;
#22363=AXIS2_PLACEMENT_3D ( 'NONE', #8946, #10861, #20032 ) ;
#22366=DIRECTION ( 'NONE',  ( 7.087422195345011518E-32, 1.000000000000000000, -0.000000000000000000 ) ) ;
#22368=FACE_BOUND ( 'NONE', #17360, .T. ) ;
#22369=ORIENTED_EDGE ( 'NONE', *, *, #23114, .F. ) ;
#22374=CARTESIAN_POINT ( 'NONE',  ( 118.3095189484530181, 10.00000000000001599, 17.50000000000003908 ) ) ;
#22379=LINE ( 'NONE', #3949, #9533 ) ;
#22389=CARTESIAN_POINT ( 'NONE',  ( 8.718769219667262149, -11.25000000000000355, 5.000000000000079936 ) ) ;
#22396=ORIENTED_EDGE ( 'NONE', *, *, #9661, .F. ) ;
#22400=EDGE_CURVE ( 'NONE', #17853, #7410, #7512, .T. ) ;
#22403=EDGE_LOOP ( 'NONE', ( #2618, #16644, #16653, #12430 ) ) ;
#22404=ADVANCED_FACE ( 'NONE', ( #22579 ), #14954, .F. ) ;
#22405=EDGE_LOOP ( 'NONE', ( #1579, #22561, #8760, #14624 ) ) ;
#22419=CARTESIAN_POINT ( 'NONE',  ( 45.00000000000000000, 2.399706452296377801, 55.00000000000021316 ) ) ;
#22424=LINE ( 'NONE', #20633, #12866 ) ;
#22425=ORIENTED_EDGE ( 'NONE', *, *, #16551, .T. ) ;
#22457=LINE ( 'NONE', #22702, #22894 ) ;
#22460=EDGE_CURVE ( 'NONE', #17999, #6426, #4842, .T. ) ;
#22463=CARTESIAN_POINT ( 'NONE',  ( 18.14354716966726144, -11.25000000000000355, 5.000000000000079936 ) ) ;
#22464=ORIENTED_EDGE ( 'NONE', *, *, #20012, .T. ) ;
#22466=AXIS2_PLACEMENT_3D ( 'NONE', #13164, #16869, #14728 ) ;
#22469=CARTESIAN_POINT ( 'NONE',  ( -11.84783529071655295, -8.974600000000002353, 5.000000000000079936 ) ) ;
#22471=CARTESIAN_POINT ( 'NONE',  ( 37.81203609676620658, -9.000000000000003553, 5.000000000000079936 ) ) ;
#22478=PLANE ( 'NONE',  #5579 ) ;
#22481=CYLINDRICAL_SURFACE ( 'NONE', #15897, 5.000000000000011546 ) ;
#22483=CARTESIAN_POINT ( 'NONE',  ( 22.71892870323381786, -9.000000000000003553, 5.000000000000079936 ) ) ;
#22492=EDGE_CURVE ( 'NONE', #7460, #13757, #12302, .T. ) ;
#22500=ORIENTED_EDGE ( 'NONE', *, *, #22940, .F. ) ;
#22503=VECTOR ( 'NONE', #21798, 1000.000000000000000 ) ;
#22509=LINE ( 'NONE', #8164, #16496 ) ;
#22516=LINE ( 'NONE', #6957, #2856 ) ;
#22523=CARTESIAN_POINT ( 'NONE',  ( 50.00000000000000000, -10.00000000000001954, 15.00000000000002842 ) ) ;
#22527=VERTEX_POINT ( 'NONE', #21230 ) ;
#22547=PLANE ( 'NONE',  #19110 ) ;
#22559=VECTOR ( 'NONE', #15772, 1000.000000000000000 ) ;
#22561=ORIENTED_EDGE ( 'NONE', *, *, #16652, .T. ) ;
#22563=EDGE_CURVE ( 'NONE', #18607, #12520, #19329, .T. ) ;
#22565=VECTOR ( 'NONE', #2354, 1000.000000000000000 ) ;
#22575=VECTOR ( 'NONE', #17172, 1000.000000000000000 ) ;
#22579=FACE_OUTER_BOUND ( 'NONE', #15976, .T. ) ;
#22582=EDGE_LOOP ( 'NONE', ( #2922, #3973, #15190, #14385 ) ) ;
#22583=PLANE ( 'NONE',  #11145 ) ;
#22587=ORIENTED_EDGE ( 'NONE', *, *, #6763, .T. ) ;
#22604=PLANE ( 'NONE',  #575 ) ;
#22605=CARTESIAN_POINT ( 'NONE',  ( 45.00000000000000000, -2.399706452296352932, 60.00000000000021316 ) ) ;
#22606=ORIENTED_EDGE ( 'NONE', *, *, #2528, .T. ) ;
#22607=LINE ( 'NONE', #17106, #763 ) ;
#22608=LINE ( 'NONE', #17472, #601 ) ;
#22610=ORIENTED_EDGE ( 'NONE', *, *, #13935, .F. ) ;
#22612=DIRECTION ( 'NONE',  ( 0.3420201433256622736, 0.9396926207859106484, 0.000000000000000000 ) ) ;
#22616=FACE_BOUND ( 'NONE', #16741, .T. ) ;
#22631=CARTESIAN_POINT ( 'NONE',  ( 40.96287359071656908, -8.974600000000002353, 5.000000000000079936 ) ) ;
#22633=ORIENTED_EDGE ( 'NONE', *, *, #13752, .T. ) ;
#22643=ORIENTED_EDGE ( 'NONE', *, *, #6439, .T. ) ;
#22644=CARTESIAN_POINT ( 'NONE',  ( -6.989194030332740226, -11.25000000000000355, 5.000000000000079936 ) ) ;
#22653=PLANE ( 'NONE',  #18364 ) ;
#22662=FACE_OUTER_BOUND ( 'NONE', #9986, .T. ) ;
#22671=ORIENTED_EDGE ( 'NONE', *, *, #20791, .F. ) ;
#22680=VECTOR ( 'NONE', #13861, 1000.000000000000114 ) ;
#22681=CARTESIAN_POINT ( 'NONE',  ( -19.99999999999999645, -9.000000000000003553, 5.000000000000079936 ) ) ;
#22689=DIRECTION ( 'NONE',  ( -4.930380657631312836E-32, -0.3420201433256691015, -0.9396926207859083169 ) ) ;
#22701=EDGE_CURVE ( 'NONE', #23136, #17296, #5318, .T. ) ;
#22702=CARTESIAN_POINT ( 'NONE',  ( -19.99999999999999645, -9.000000000000003553, 5.000000000000079936 ) ) ;
#22703=ADVANCED_FACE ( 'NONE', ( #9051 ), #22547, .F. ) ;
#22704=AXIS2_PLACEMENT_3D ( 'NONE', #8216, #10028, #6411 ) ;
#22722=ORIENTED_EDGE ( 'NONE', *, *, #15139, .T. ) ;
#22725=CARTESIAN_POINT ( 'NONE',  ( 49.55947366966726264, -11.25000000000000355, 5.000000000000079936 ) ) ;
#22729=ORIENTED_EDGE ( 'NONE', *, *, #3220, .T. ) ;
#22731=VERTEX_POINT ( 'NONE', #22297 ) ;
#22738=DIRECTION ( 'NONE',  ( 0.000000000000000000, 0.000000000000000000, 1.000000000000000000 ) ) ;
#22746=VECTOR ( 'NONE', #15456, 1000.000000000000000 ) ;
#22748=VERTEX_POINT ( 'NONE', #7727 ) ;
#22750=DIRECTION ( 'NONE',  ( 7.087422195345011518E-32, 1.000000000000000000, -0.000000000000000000 ) ) ;
#22755=LINE ( 'NONE', #15249, #15145 ) ;
#22764=CARTESIAN_POINT ( 'NONE',  ( 45.00000000000000000, 10.00000000000001599, 15.00000000000003020 ) ) ;
#22778=CARTESIAN_POINT ( 'NONE',  ( 46.41788101966725577, -11.25000000000000355, 5.000000000000079936 ) ) ;
#22779=VERTEX_POINT ( 'NONE', #3742 ) ;
#22798=EDGE_CURVE ( 'NONE', #20481, #15099, #15275, .T. ) ;
#22801=DIRECTION ( 'NONE',  ( 1.000000000000000000, 7.703719777548943412E-32, 0.000000000000000000 ) ) ;
#22805=EDGE_CURVE ( 'NONE', #2366, #633, #4108, .T. ) ;
#22810=EDGE_LOOP ( 'NONE', ( #20359, #13527, #371, #4790 ) ) ;
#22814=ORIENTED_EDGE ( 'NONE', *, *, #16134, .F. ) ;
#22819=EDGE_CURVE ( 'NONE', #16967, #22748, #18838, .T. ) ;
#22824=ORIENTED_EDGE ( 'NONE', *, *, #11628, .T. ) ;
#22836=CARTESIAN_POINT ( 'NONE',  ( 3.851282720981234142, -0.3188430404951885788, 10.00000000000008882 ) ) ;
#22837=DIRECTION ( 'NONE',  ( 1.000000000000000000, 7.703719777548943412E-32, 0.000000000000000000 ) ) ;
#22838=CARTESIAN_POINT ( 'NONE',  ( -19.99999999999999645, -11.25000000000000355, 10.00000000000008882 ) ) ;
#22839=VECTOR ( 'NONE', #19340, 1000.000000000000114 ) ;
#22860=EDGE_CURVE ( 'NONE', #18371, #313, #11326, .T. ) ;
#22868=LINE ( 'NONE', #4908, #7118 ) ;
#22871=ORIENTED_EDGE ( 'NONE', *, *, #753, .T. ) ;
#22879=VERTEX_POINT ( 'NONE', #13942 ) ;
#22886=PLANE ( 'NONE',  #8709 ) ;
#22887=DIRECTION ( 'NONE',  ( -1.000000000000000000, -7.703719777548943412E-32, 0.000000000000000000 ) ) ;
#22894=VECTOR ( 'NONE', #19118, 1000.000000000000000 ) ;
#22898=DIRECTION ( 'NONE',  ( -1.000000000000000000, -7.703719777548943412E-32, 0.000000000000000000 ) ) ;
#22899=ORIENTED_EDGE ( 'NONE', *, *, #20765, .F. ) ;
#22900=DIRECTION ( 'NONE',  ( 0.000000000000000000, 0.000000000000000000, -1.000000000000000000 ) ) ;
#22909=EDGE_CURVE ( 'NONE', #15108, #23499, #6624, .T. ) ;
#22938=ORIENTED_EDGE ( 'NONE', *, *, #13669, .F. ) ;
#22940=EDGE_CURVE ( 'NONE', #12921, #18952, #13587, .T. ) ;
#22944=ORIENTED_EDGE ( 'NONE', *, *, #2470, .F. ) ;
#22953=ORIENTED_EDGE ( 'NONE', *, *, #12623, .F. ) ;
#22960=ORIENTED_EDGE ( 'NONE', *, *, #14104, .F. ) ;
#22961=LINE ( 'NONE', #9698, #17616 ) ;
#22970=EDGE_CURVE ( 'NONE', #5149, #15108, #4460, .T. ) ;
#22972=ORIENTED_EDGE ( 'NONE', *, *, #17089, .F. ) ;
#22974=ORIENTED_EDGE ( 'NONE', *, *, #23226, .T. ) ;
#22985=FACE_OUTER_BOUND ( 'NONE', #8265, .T. ) ;
#22988=CARTESIAN_POINT ( 'NONE',  ( 7.829898480332751376, -11.25000000000000355, 5.000000000000079936 ) ) ;
#23003=ORIENTED_EDGE ( 'NONE', *, *, #9496, .T. ) ;
#23005=VERTEX_POINT ( 'NONE', #15396 ) ;
#23008=EDGE_CURVE ( 'NONE', #2702, #11449, #18951, .T. ) ;
#23009=DIRECTION ( 'NONE',  ( -0.9396926207859107594, -0.3420201433256623291, 1.540743955509804830E-32 ) ) ;
#23019=CARTESIAN_POINT ( 'NONE',  ( -14.16125006966725053, -11.25000000000000355, 5.000000000000079936 ) ) ;
#23026=ORIENTED_EDGE ( 'NONE', *, *, #3169, .T. ) ;
#23034=CARTESIAN_POINT ( 'NONE',  ( 14.94766720513313096, 3.719910619709361654, 10.00000000000008882 ) ) ;
#23035=FACE_OUTER_BOUND ( 'NONE', #3446, .T. ) ;
#23050=DIRECTION ( 'NONE',  ( 0.3420201433256622181, 0.9396926207859107594, -6.162975822039141593E-32 ) ) ;
#23053=ORIENTED_EDGE ( 'NONE', *, *, #21516, .T. ) ;
#23056=ORIENTED_EDGE ( 'NONE', *, *, #23156, .T. ) ;
#23069=DIRECTION ( 'NONE',  ( -0.9396926207859107594, -0.3420201433256623291, 1.540743955509804830E-32 ) ) ;
#23077=CARTESIAN_POINT ( 'NONE',  ( 37.82128094071656932, -8.974600000000002353, 10.00000000000008882 ) ) ;
#23079=DIRECTION ( 'NONE',  ( 7.010384997569516610E-32, 1.000000000000000000, -3.469446951953615175E-16 ) ) ;
#23081=LINE ( 'NONE', #8382, #18700 ) ;
#23082=ORIENTED_EDGE ( 'NONE', *, *, #2461, .T. ) ;
#23089=EDGE_CURVE ( 'NONE', #3670, #14717, #17408, .T. ) ;
#23101=EDGE_CURVE ( 'NONE', #2869, #4263, #17756, .T. ) ;
#23110=EDGE_LOOP ( 'NONE', ( #5620, #9609, #21416, #19195 ) ) ;
#23113=DIRECTION ( 'NONE',  ( 1.000000000000000000, 7.703719777548943412E-32, 0.000000000000000000 ) ) ;
#23114=EDGE_CURVE ( 'NONE', #8738, #10010, #9028, .T. ) ;
#23131=ORIENTED_EDGE ( 'NONE', *, *, #9134, .F. ) ;
#23136=VERTEX_POINT ( 'NONE', #18104 ) ;
#23146=CARTESIAN_POINT ( 'NONE',  ( 3.254516946766198959, -9.000000000000003553, 5.000000000000079936 ) ) ;
#23156=EDGE_CURVE ( 'NONE', #19783, #10249, #14048, .T. ) ;
#23161=CARTESIAN_POINT ( 'NONE',  ( 22.10407284676620066, -9.000000000000001776, 10.00000000000008882 ) ) ;
#23162=ORIENTED_EDGE ( 'NONE', *, *, #21069, .F. ) ;
#23165=VERTEX_POINT ( 'NONE', #18219 ) ;
#23167=AXIS2_PLACEMENT_3D ( 'NONE', #3081, #6925, #14242 ) ;
#23183=CARTESIAN_POINT ( 'NONE',  ( 5.577176569667260608, -11.25000000000000355, 10.00000000000008882 ) ) ;
#23189=CARTESIAN_POINT ( 'NONE',  ( 14.11308378033275446, -11.25000000000000355, 5.000000000000079936 ) ) ;
#23191=CARTESIAN_POINT ( 'NONE',  ( 10.14331325928345073, -8.974600000000002353, 5.000000000000079936 ) ) ;
#23192=ORIENTED_EDGE ( 'NONE', *, *, #2371, .F. ) ;
#23204=FACE_OUTER_BOUND ( 'NONE', #11421, .T. ) ;
#23208=DIRECTION ( 'NONE',  ( 0.3420201433256622181, 0.9396926207859107594, -6.162975822039141593E-32 ) ) ;
#23217=DIRECTION ( 'NONE',  ( 0.000000000000000000, 0.000000000000000000, 1.000000000000000000 ) ) ;
#23226=EDGE_CURVE ( 'NONE', #19389, #7167, #10475, .T. ) ;
#23227=EDGE_LOOP ( 'NONE', ( #7412, #17528, #4213, #14267 ) ) ;
#23236=DIRECTION ( 'NONE',  ( -1.000000000000000000, -7.703719777548943412E-32, 0.000000000000000000 ) ) ;
#23238=VECTOR ( 'NONE', #21541, 1000.000000000000000 ) ;
#23247=LINE ( 'NONE', #19895, #18521 ) ;
#23248=ORIENTED_EDGE ( 'NONE', *, *, #9360, .F. ) ;
#23254=LINE ( 'NONE', #1216, #21224 ) ;
#23258=ADVANCED_FACE ( 'NONE', ( #21438 ), #5052, .T. ) ;
#23260=CARTESIAN_POINT ( 'NONE',  ( 47.24605889071655440, -8.974600000000002353, 5.000000000000079936 ) ) ;
#23263=VECTOR ( 'NONE', #20217, 1000.000000000000000 ) ;
#23267=EDGE_CURVE ( 'NONE', #4326, #3825, #14772, .T. ) ;
#23269=CARTESIAN_POINT ( 'NONE',  ( -19.99999999999999645, -11.25000000000000355, 5.000000000000079936 ) ) ;
#23284=ORIENTED_EDGE ( 'NONE', *, *, #10165, .F. ) ;
#23287=PLANE ( 'NONE',  #22363 ) ;
#23288=VERTEX_POINT ( 'NONE', #4203 ) ;
#23296=CIRCLE ( 'NONE', #15294, 1.000000000000002665 ) ;
#23302=ADVANCED_FACE ( 'NONE', ( #7574 ), #2398, .F. ) ;
#23317=FACE_OUTER_BOUND ( 'NONE', #5356, .T. ) ;
#23318=CARTESIAN_POINT ( 'NONE',  ( 13.28490590928345405, -8.974600000000002353, 5.000000000000079936 ) ) ;
#23329=AXIS2_PLACEMENT_3D ( 'NONE', #16435, #11056, #4080 ) ;
#23333=LINE ( 'NONE', #84, #2963 ) ;
#23334=DIRECTION ( 'NONE',  ( 0.3420201433256622736, -0.9396926207859106484, -1.232595164407828100E-31 ) ) ;
#23345=EDGE_LOOP ( 'NONE', ( #12493, #5087, #16995, #14579, #6978, #11969, #3354, #20394, #17562, #496, #15808, #22606, #7067, #15454, #2040, #10098, #12309, #14658, #22974, #17757, #3883, #14551, #5381, #1364, #12349, #23053, #19056, #15102, #16706, #5895, #13895, #13181, #18457, #11609, #21566, #9476, #7046, #17737, #19592, #8724, #11331, #5847, #3668, #3637, #13520, #4917, #1124, #6209, #20542, #8856, #7607, #5831, #7383, #9688, #21420, #11456, #5001, #14259, #104, #29, #11030, #6034, #10159, #6156, #19144, #19425, #7728, #19539, #4053, #8383, #19635, #201, #20479, #17661, #20505, #14425, #13043, #4775, #21973, #12247, #4060, #12388, #627, #6923, #14570, #19546, #7235, #19230, #11891, #3823, #10162, #2814, #20814 ) ) ;
#23353=LINE ( 'NONE', #12249, #21959 ) ;
#23359=ORIENTED_EDGE ( 'NONE', *, *, #14816, .T. ) ;
#23365=CARTESIAN_POINT ( 'NONE',  ( -13.27237933033274153, -11.25000000000000355, 10.00000000000008882 ) ) ;
#23371=PLANE ( 'NONE',  #6911 ) ;
#23375=ORIENTED_EDGE ( 'NONE', *, *, #8101, .T. ) ;
#23391=PLANE ( 'NONE',  #6072 ) ;
#23402=LINE ( 'NONE', #3159, #21269 ) ;
#23409=DIRECTION ( 'NONE',  ( 0.000000000000000000, 0.000000000000000000, -1.000000000000000000 ) ) ;
#23410=ORIENTED_EDGE ( 'NONE', *, *, #7030, .T. ) ;
#23413=VERTEX_POINT ( 'NONE', #9621 ) ;
#23419=PLANE ( 'NONE',  #6407 ) ;
#23431=CARTESIAN_POINT ( 'NONE',  ( 26.04405168928502334, 7.758664279913913830, 10.00000000000008882 ) ) ;
#23432=CARTESIAN_POINT ( 'NONE',  ( 34.67044344676619971, -9.000000000000007105, 5.000000000000079936 ) ) ;
#23437=EDGE_CURVE ( 'NONE', #15099, #2752, #13209, .T. ) ;
#23448=CARTESIAN_POINT ( 'NONE',  ( 45.00000000000000000, 10.00000000000001599, 34.11836509645781490 ) ) ;
#23451=ORIENTED_EDGE ( 'NONE', *, *, #18323, .T. ) ;
#23454=CARTESIAN_POINT ( 'NONE',  ( -19.99999999999999645, -9.000000000000003553, 5.000000000000079936 ) ) ;
#23458=DIRECTION ( 'NONE',  ( 0.000000000000000000, 0.000000000000000000, 1.000000000000000000 ) ) ;
#23459=ORIENTED_EDGE ( 'NONE', *, *, #11731, .F. ) ;
#23466=ORIENTED_EDGE ( 'NONE', *, *, #23602, .F. ) ;
#23472=ORIENTED_EDGE ( 'NONE', *, *, #8196, .T. ) ;
#23476=LINE ( 'NONE', #19987, #11490 ) ;
#23482=( BOUNDED_CURVE ( )  B_SPLINE_CURVE ( 3, ( #17092, #664, #15322, #16973 ),
 .UNSPECIFIED., .F., .F. ) 
 B_SPLINE_CURVE_WITH_KNOTS ( ( 4, 4 ),
 ( 1.570796326794896558, 1.666162211095538082 ),
 .UNSPECIFIED. ) 
 CURVE ( )  GEOMETRIC_REPRESENTATION_ITEM ( )  RATIONAL_B_SPLINE_CURVE ( ( 1.000000000000000000, 0.9992422559301721297, 0.9992422559301721297, 1.000000000000000000 ) ) 
 REPRESENTATION_ITEM ( '' )  );
#23489=CARTESIAN_POINT ( 'NONE',  ( 49.55947366966726264, -11.25000000000000355, 5.000000000000079936 ) ) ;
#23490=ORIENTED_EDGE ( 'NONE', *, *, #6855, .F. ) ;
#23495=DIRECTION ( 'NONE',  ( -0.3420201433256622181, 0.9396926207859106484, 1.232595164407828100E-31 ) ) ;
#23499=VERTEX_POINT ( 'NONE', #8056 ) ;
#23504=VECTOR ( 'NONE', #8050, 1000.000000000000000 ) ;
#23509=FACE_OUTER_BOUND ( 'NONE', #12015, .T. ) ;
#23511=DIRECTION ( 'NONE',  ( -1.000000000000000000, -7.703719777548943412E-32, 0.000000000000000000 ) ) ;
#23520=VECTOR ( 'NONE', #21417, 1000.000000000000000 ) ;
#23525=ORIENTED_EDGE ( 'NONE', *, *, #11990, .F. ) ;
#23529=CARTESIAN_POINT ( 'NONE',  ( 3.869372803233808611, -9.000000000000001776, 10.00000000000008882 ) ) ;
#23530=PLANE ( 'NONE',  #19053 ) ;
#23531=ORIENTED_EDGE ( 'NONE', *, *, #2796, .T. ) ;
#23541=EDGE_CURVE ( 'NONE', #1835, #4715, #4439, .T. ) ;
#23548=CARTESIAN_POINT ( 'NONE',  ( -12.45344630323380031, -9.000000000000003553, 5.000000000000079936 ) ) ;
#23549=VECTOR ( 'NONE', #13535, 1000.000000000000000 ) ;
#23551=CARTESIAN_POINT ( 'NONE',  ( 7.010965453233809264, -9.000000000000001776, 5.000000000000079936 ) ) ;
#23553=LINE ( 'NONE', #10536, #1142 ) ;
#23556=VERTEX_POINT ( 'NONE', #15370 ) ;
#23563=ORIENTED_EDGE ( 'NONE', *, *, #18619, .T. ) ;
#23569=DIRECTION ( 'NONE',  ( -1.000000000000000000, -7.703719777548943412E-32, 0.000000000000000000 ) ) ;
#23578=FACE_OUTER_BOUND ( 'NONE', #10394, .T. ) ;
#23581=LINE ( 'NONE', #7191, #8870 ) ;
#23582=ORIENTED_EDGE ( 'NONE', *, *, #7023, .T. ) ;
#23587=CARTESIAN_POINT ( 'NONE',  ( 28.38725814676620018, -9.000000000000003553, 5.000000000000079936 ) ) ;
#23602=EDGE_CURVE ( 'NONE', #12158, #17853, #17380, .T. ) ;
#23604=CARTESIAN_POINT ( 'NONE',  ( 45.00000000000000000, -14.69846310392956745, 35.82846581308617573 ) ) ;
#23622=VECTOR ( 'NONE', #17455, 1000.000000000000114 ) ;
#23623=ORIENTED_EDGE ( 'NONE', *, *, #15954, .F. ) ;
#23638=LINE ( 'NONE', #6887, #1254 ) ;
#23641=FACE_OUTER_BOUND ( 'NONE', #11582, .T. ) ;
#23649=ORIENTED_EDGE ( 'NONE', *, *, #270, .T. ) ;
#23650=AXIS2_PLACEMENT_3D ( 'NONE', #15585, #10075, #11988 ) ;
#23651=CARTESIAN_POINT ( 'NONE',  ( -19.99999999999999645, -15.00000000000001954, 5.000000000000079936 ) ) ;
#23652=DIRECTION ( 'NONE',  ( 0.000000000000000000, 0.000000000000000000, 1.000000000000000000 ) ) ;
#23653=ORIENTED_EDGE ( 'NONE', *, *, #6862, .T. ) ;
#23656=VECTOR ( 'NONE', #21261, 1000.000000000000114 ) ;
#23667=EDGE_CURVE ( 'NONE', #12703, #15725, #12482, .T. ) ;
#23675=ORIENTED_EDGE ( 'NONE', *, *, #9830, .T. ) ;
#23679=EDGE_CURVE ( 'NONE', #19575, #9029, #17626, .T. ) ;
#23681=ORIENTED_EDGE ( 'NONE', *, *, #15861, .F. ) ;
#23693=CARTESIAN_POINT ( 'NONE',  ( 18.96248019676619734, -9.000000000000003553, 5.000000000000079936 ) ) ;
#23695=LINE ( 'NONE', #16746, #6173 ) ;
ENDSEC;
END-ISO-10303-21;
